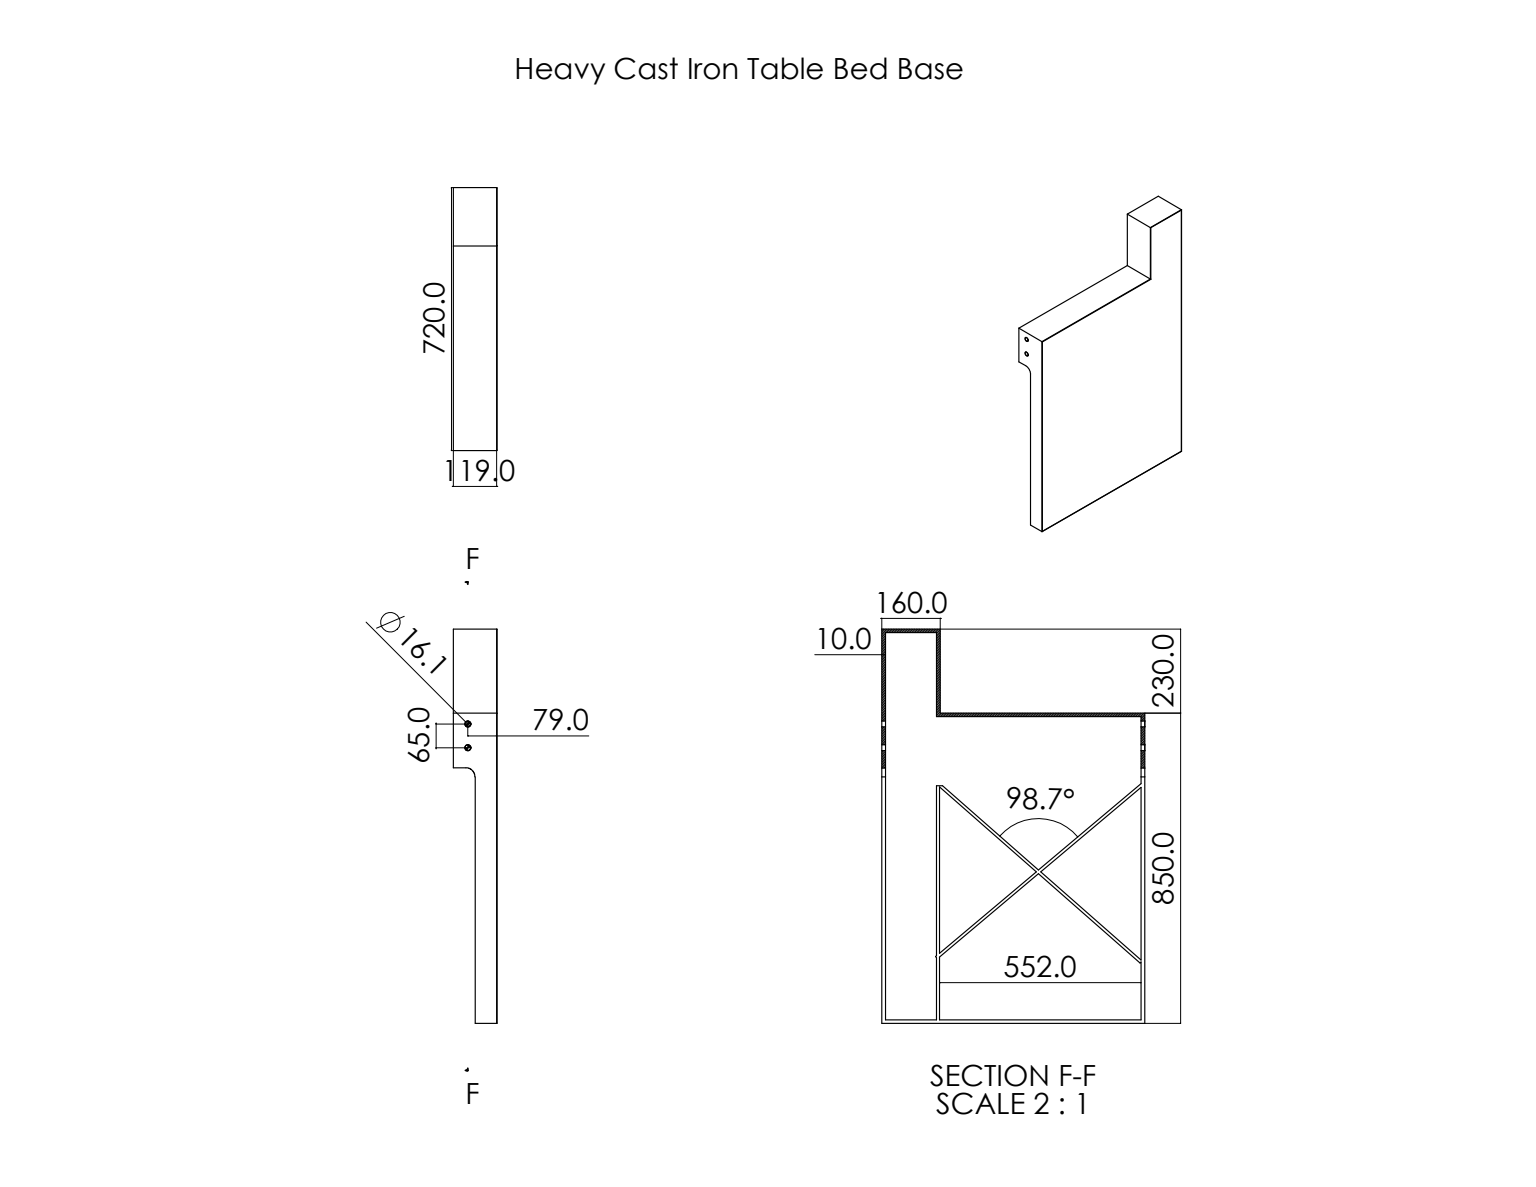
ISO-10303-21;
HEADER;
FILE_DESCRIPTION (('STEP AP214'),
    '1' );
FILE_NAME ('Heavy Cast Iron Table Bed Base.step',
    '2026-10-21T17:07:05',
    ( '' ),
    ( '' ),
    'SwSTEP 2.0',
    'SolidWorks 2025',
    '' );
FILE_SCHEMA (( 'AUTOMOTIVE_DESIGN' ));
ENDSEC;

DATA;
#65=ORIENTED_EDGE ( 'NONE', *, *, #36847, .T. ) ;
#80=ORIENTED_EDGE ( 'NONE', *, *, #38468, .F. ) ;
#82=DIRECTION ( 'NONE',  ( -0.000000000000000000, -1.000000000000000000, -0.000000000000000000 ) ) ;
#112=ORIENTED_EDGE ( 'NONE', *, *, #9772, .T. ) ;
#118=LINE ( 'NONE', #10283, #45262 ) ;
#145=CARTESIAN_POINT ( 'NONE',  ( 187.1337867209877857, 56.73212367640085318, 362.5753187112032379 ) ) ;
#155=DIRECTION ( 'NONE',  ( 0.000000000000000000, 0.000000000000000000, 1.000000000000000000 ) ) ;
#178=VECTOR ( 'NONE', #201, 1000.000000000000114 ) ;
#195=DIRECTION ( 'NONE',  ( 0.000000000000000000, -1.000000000000000000, 1.672022627447525240E-16 ) ) ;
#201=DIRECTION ( 'NONE',  ( -1.236450975029139710E-16, 0.7517448203044212462, 0.6594541114781782287 ) ) ;
#267=( BOUNDED_CURVE ( )  B_SPLINE_CURVE ( 3, ( #30983, #13892, #3032, #6720 ),
 .UNSPECIFIED., .F., .T. ) 
 B_SPLINE_CURVE_WITH_KNOTS ( ( 4, 4 ),
 ( 1.570796326794896558, 3.141592653589793116 ),
 .UNSPECIFIED. ) 
 CURVE ( )  GEOMETRIC_REPRESENTATION_ITEM ( )  RATIONAL_B_SPLINE_CURVE ( ( 1.000000000000000000, 0.8047378541243649375, 0.8047378541243649375, 1.000000000000000000 ) ) 
 REPRESENTATION_ITEM ( '' )  );
#273=CARTESIAN_POINT ( 'NONE',  ( 879.9999999999992042, 479.9999999999998863, -210.0000000000000000 ) ) ;
#291=AXIS2_PLACEMENT_3D ( 'NONE', #13040, #41443, #41905 ) ;
#352=EDGE_CURVE ( 'NONE', #861, #2741, #13234, .T. ) ;
#354=ORIENTED_EDGE ( 'NONE', *, *, #13193, .T. ) ;
#359=AXIS2_PLACEMENT_3D ( 'NONE', #31798, #9874, #27892 ) ;
#366=VECTOR ( 'NONE', #18473, 1000.000000000000000 ) ;
#377=DIRECTION ( 'NONE',  ( 0.000000000000000000, -0.6594541114781790059, 0.7517448203044204691 ) ) ;
#407=ORIENTED_EDGE ( 'NONE', *, *, #12306, .F. ) ;
#449=ADVANCED_FACE ( 'NONE', ( #27988 ), #38617, .F. ) ;
#535=EDGE_LOOP ( 'NONE', ( #2161, #41639, #39801, #23830 ) ) ;
#545=ORIENTED_EDGE ( 'NONE', *, *, #45289, .F. ) ;
#562=VECTOR ( 'NONE', #15359, 1000.000000000000000 ) ;
#623=DIRECTION ( 'NONE',  ( -0.000000000000000000, -0.000000000000000000, 1.000000000000000000 ) ) ;
#624=CARTESIAN_POINT ( 'NONE',  ( 999.9999999999992042, 239.9999999999998863, -209.9999999999999716 ) ) ;
#642=ORIENTED_EDGE ( 'NONE', *, *, #31723, .T. ) ;
#658=AXIS2_PLACEMENT_3D ( 'NONE', #4761, #18865, #32956 ) ;
#660=CARTESIAN_POINT ( 'NONE',  ( 989.9999999999992042, 62.79977829742938411, -207.3621835540872951 ) ) ;
#693=EDGE_CURVE ( 'NONE', #4054, #5516, #21293, .T. ) ;
#779=LINE ( 'NONE', #28956, #941 ) ;
#782=PLANE ( 'NONE',  #39472 ) ;
#802=CARTESIAN_POINT ( 'NONE',  ( 939.9999999999992042, 50.81038600091411439, -209.9999999999999716 ) ) ;
#826=DIRECTION ( 'NONE',  ( 1.000000000000000000, 0.000000000000000000, 0.000000000000000000 ) ) ;
#831=DIRECTION ( 'NONE',  ( 1.000000000000000000, -0.000000000000000000, 0.000000000000000000 ) ) ;
#849=EDGE_LOOP ( 'NONE', ( #8777, #12953, #44083, #25218 ) ) ;
#861=VERTEX_POINT ( 'NONE', #21514 ) ;
#884=( GEOMETRIC_REPRESENTATION_CONTEXT ( 3 ) GLOBAL_UNCERTAINTY_ASSIGNED_CONTEXT ( ( #29214 ) ) GLOBAL_UNIT_ASSIGNED_CONTEXT ( ( #30081, #19913, #9523 ) ) REPRESENTATION_CONTEXT ( 'NONE', 'WORKASPACE' ) );
#887=DIRECTION ( 'NONE',  ( 1.000000000000000000, -0.000000000000000000, -0.000000000000000000 ) ) ;
#920=EDGE_LOOP ( 'NONE', ( #2986, #31243, #45604, #112 ) ) ;
#937=CYLINDRICAL_SURFACE ( 'NONE', #26687, 1.000000000000000888 ) ;
#941=VECTOR ( 'NONE', #28498, 1000.000000000000000 ) ;
#960=EDGE_CURVE ( 'NONE', #27431, #8959, #32146, .T. ) ;
#966=VERTEX_POINT ( 'NONE', #41454 ) ;
#985=LINE ( 'NONE', #15090, #37294 ) ;
#1013=VECTOR ( 'NONE', #42593, 1000.000000000000000 ) ;
#1015=LINE ( 'NONE', #7286, #17369 ) ;
#1032=VERTEX_POINT ( 'NONE', #9806 ) ;
#1086=ORIENTED_EDGE ( 'NONE', *, *, #38685, .T. ) ;
#1104=DIRECTION ( 'NONE',  ( 0.000000000000000000, 0.7517448203044204691, 0.6594541114781790059 ) ) ;
#1115=AXIS2_PLACEMENT_3D ( 'NONE', #34295, #31290, #10275 ) ;
#1184=VECTOR ( 'NONE', #2168, 1000.000000000000000 ) ;
#1224=DIRECTION ( 'NONE',  ( -0.000000000000000000, -0.000000000000000000, -1.000000000000000000 ) ) ;
#1258=ADVANCED_FACE ( 'NONE', ( #30594 ), #30141, .T. ) ;
#1274=AXIS2_PLACEMENT_3D ( 'NONE', #17291, #20745, #24904 ) ;
#1308=CARTESIAN_POINT ( 'NONE',  ( 1820.038553321469863, -407.8586036264140375, -201.9999999999998863 ) ) ;
#1332=LINE ( 'NONE', #25597, #4420 ) ;
#1340=PLANE ( 'NONE',  #41833 ) ;
#1354=ORIENTED_EDGE ( 'NONE', *, *, #44887, .F. ) ;
#1358=LINE ( 'NONE', #15461, #15140 ) ;
#1397=CARTESIAN_POINT ( 'NONE',  ( 989.9999999999992042, 249.9999999999998863, 350.0000000000000000 ) ) ;
#1451=CARTESIAN_POINT ( 'NONE',  ( 914.9999999999992042, 99.99999999999984368, -350.0000000000000000 ) ) ;
#1463=FACE_OUTER_BOUND ( 'NONE', #20948, .T. ) ;
#1488=ORIENTED_EDGE ( 'NONE', *, *, #32844, .T. ) ;
#1513=DIRECTION ( 'NONE',  ( -1.058954862565134068E-16, 0.6438296778008191223, 0.7651688349527137056 ) ) ;
#1543=ADVANCED_FACE ( 'NONE', ( #10261 ), #24338, .F. ) ;
#1561=EDGE_CURVE ( 'NONE', #38354, #16465, #40038, .T. ) ;
#1599=EDGE_LOOP ( 'NONE', ( #39442, #9325, #33134, #32362 ) ) ;
#1601=DIRECTION ( 'NONE',  ( 0.000000000000000000, 0.7651688349527167032, -0.6438296778008156807 ) ) ;
#1678=CARTESIAN_POINT ( 'NONE',  ( 187.1337867209877857, -422.8782571739196783, -207.4246812887968190 ) ) ;
#1680=ORIENTED_EDGE ( 'NONE', *, *, #36506, .F. ) ;
#1729=( BOUNDED_CURVE ( )  B_SPLINE_CURVE ( 3, ( #32757, #8061, #36212, #40382 ),
 .UNSPECIFIED., .F., .T. ) 
 B_SPLINE_CURVE_WITH_KNOTS ( ( 4, 4 ),
 ( 4.712388980384689674, 6.283185307179586232 ),
 .UNSPECIFIED. ) 
 CURVE ( )  GEOMETRIC_REPRESENTATION_ITEM ( )  RATIONAL_B_SPLINE_CURVE ( ( 1.000000000000000000, 0.8047378541243649375, 0.8047378541243649375, 1.000000000000000000 ) ) 
 REPRESENTATION_ITEM ( '' )  );
#1751=AXIS2_PLACEMENT_3D ( 'NONE', #40538, #8887, #9347 ) ;
#1773=LINE ( 'NONE', #45441, #7634 ) ;
#1842=FACE_OUTER_BOUND ( 'NONE', #3408, .T. ) ;
#1846=EDGE_CURVE ( 'NONE', #22430, #39622, #19023, .T. ) ;
#1907=AXIS2_PLACEMENT_3D ( 'NONE', #37509, #40532, #8881 ) ;
#1920=DIRECTION ( 'NONE',  ( 1.000000000000000000, 0.000000000000000000, 0.000000000000000000 ) ) ;
#1935=DIRECTION ( 'NONE',  ( 0.000000000000000000, 0.000000000000000000, 1.000000000000000000 ) ) ;
#1941=ORIENTED_EDGE ( 'NONE', *, *, #25313, .F. ) ;
#1951=CARTESIAN_POINT ( 'NONE',  ( 999.9999999999992042, -600.0000000000001137, 359.0000000000000000 ) ) ;
#1973=CARTESIAN_POINT ( 'NONE',  ( 1820.038553321469863, -418.3138125091624602, -201.9999999999998863 ) ) ;
#1975=ORIENTED_EDGE ( 'NONE', *, *, #8593, .F. ) ;
#1989=ORIENTED_EDGE ( 'NONE', *, *, #19944, .T. ) ;
#2055=ORIENTED_EDGE ( 'NONE', *, *, #24398, .F. ) ;
#2059=FACE_BOUND ( 'NONE', #7636, .T. ) ;
#2079=EDGE_CURVE ( 'NONE', #40848, #12356, #33501, .T. ) ;
#2113=ORIENTED_EDGE ( 'NONE', *, *, #11760, .T. ) ;
#2156=ADVANCED_FACE ( 'NONE', ( #6514 ), #3046, .F. ) ;
#2157=ORIENTED_EDGE ( 'NONE', *, *, #14016, .F. ) ;
#2161=ORIENTED_EDGE ( 'NONE', *, *, #35912, .F. ) ;
#2168=DIRECTION ( 'NONE',  ( -0.000000000000000000, -0.000000000000000000, 1.000000000000000000 ) ) ;
#2197=LINE ( 'NONE', #41236, #38683 ) ;
#2201=CARTESIAN_POINT ( 'NONE',  ( 914.9999999999992042, 99.99999999999984368, 360.0000000000000000 ) ) ;
#2230=DIRECTION ( 'NONE',  ( 0.7071067811857625340, 0.000000000000000000, 0.7071067811873326114 ) ) ;
#2244=FACE_BOUND ( 'NONE', #18507, .T. ) ;
#2279=CARTESIAN_POINT ( 'NONE',  ( 989.9999999999992042, -590.0000000000001137, 360.0000000000000000 ) ) ;
#2345=DIRECTION ( 'NONE',  ( 1.000000000000000000, 0.000000000000000000, 0.000000000000000000 ) ) ;
#2365=ORIENTED_EDGE ( 'NONE', *, *, #4735, .T. ) ;
#2373=DIRECTION ( 'NONE',  ( 1.000000000000000000, 0.000000000000000000, -0.000000000000000000 ) ) ;
#2389=CARTESIAN_POINT ( 'NONE',  ( 939.9999999999993179, -590.0000000000001137, -209.9999999999999716 ) ) ;
#2407=VECTOR ( 'NONE', #30135, 1000.000000000000000 ) ;
#2444=ORIENTED_EDGE ( 'NONE', *, *, #21048, .F. ) ;
#2582=EDGE_CURVE ( 'NONE', #39622, #45702, #32793, .T. ) ;
#2584=LINE ( 'NONE', #16687, #20282 ) ;
#2611=CARTESIAN_POINT ( 'NONE',  ( 927.9999999999992042, 219.9999999999998863, -350.0000000000000000 ) ) ;
#2630=ADVANCED_FACE ( 'NONE', ( #36510 ), #4432, .T. ) ;
#2653=VECTOR ( 'NONE', #14168, 1000.000000000000000 ) ;
#2657=VECTOR ( 'NONE', #35418, 1000.000000000000000 ) ;
#2664=FACE_OUTER_BOUND ( 'NONE', #17522, .T. ) ;
#2693=CARTESIAN_POINT ( 'NONE',  ( 939.9999999999993179, -600.0000000000001137, -360.0000000000000000 ) ) ;
#2707=AXIS2_PLACEMENT_3D ( 'NONE', #35758, #1104, #14761 ) ;
#2741=VERTEX_POINT ( 'NONE', #23318 ) ;
#2742=ORIENTED_EDGE ( 'NONE', *, *, #25270, .T. ) ;
#2766=AXIS2_PLACEMENT_3D ( 'NONE', #23148, #37257, #2373 ) ;
#2826=LINE ( 'NONE', #36640, #40486 ) ;
#2830=DIRECTION ( 'NONE',  ( 0.000000000000000000, -1.000000000000000000, 0.000000000000000000 ) ) ;
#2888=DIRECTION ( 'NONE',  ( 0.000000000000000000, 0.000000000000000000, -1.000000000000000000 ) ) ;
#2960=ADVANCED_FACE ( 'NONE', ( #1842 ), #27635, .F. ) ;
#2986=ORIENTED_EDGE ( 'NONE', *, *, #41717, .T. ) ;
#2996=CARTESIAN_POINT ( 'NONE',  ( 914.9999999999992042, 74.99999999999984368, 350.0000000000000000 ) ) ;
#3032=CARTESIAN_POINT ( 'NONE',  ( 999.5857864376259840, 249.9999999999998863, -199.9999999999999432 ) ) ;
#3046=CYLINDRICAL_SURFACE ( 'NONE', #13598, 7.999999999999896083 ) ;
#3074=EDGE_LOOP ( 'NONE', ( #11565, #26546, #9323, #31356 ) ) ;
#3116=ORIENTED_EDGE ( 'NONE', *, *, #41125, .T. ) ;
#3147=DIRECTION ( 'NONE',  ( 0.000000000000000000, -1.000000000000000000, 0.000000000000000000 ) ) ;
#3183=ORIENTED_EDGE ( 'NONE', *, *, #16214, .F. ) ;
#3243=EDGE_LOOP ( 'NONE', ( #545, #41841, #11943 ) ) ;
#3252=ORIENTED_EDGE ( 'NONE', *, *, #8593, .T. ) ;
#3269=EDGE_CURVE ( 'NONE', #13352, #14381, #34673, .T. ) ;
#3311=AXIS2_PLACEMENT_3D ( 'NONE', #15950, #12699, #30032 ) ;
#3321=EDGE_LOOP ( 'NONE', ( #37502, #19598 ) ) ;
#3364=DIRECTION ( 'NONE',  ( 0.000000000000000000, 0.000000000000000000, 1.000000000000000000 ) ) ;
#3381=LINE ( 'NONE', #6608, #24751 ) ;
#3404=VECTOR ( 'NONE', #7997, 1000.000000000000000 ) ;
#3405=DIRECTION ( 'NONE',  ( -0.7071067811857625340, 8.659560562345319848E-17, 0.7071067811873326114 ) ) ;
#3408=EDGE_LOOP ( 'NONE', ( #13481, #19468, #22043, #26306 ) ) ;
#3413=FACE_OUTER_BOUND ( 'NONE', #849, .T. ) ;
#3424=CARTESIAN_POINT ( 'NONE',  ( 999.9999999999992042, -599.5857864376268935, -359.5857864376268935 ) ) ;
#3430=AXIS2_PLACEMENT_3D ( 'NONE', #8557, #4189, #19171 ) ;
#3548=ORIENTED_EDGE ( 'NONE', *, *, #352, .T. ) ;
#3573=EDGE_CURVE ( 'NONE', #13352, #40320, #25375, .T. ) ;
#3619=ORIENTED_EDGE ( 'NONE', *, *, #13436, .F. ) ;
#3663=PRODUCT_CONTEXT ( 'NONE', #30200, 'mechanical' ) ;
#3676=CARTESIAN_POINT ( 'NONE',  ( 939.9999999999992042, 62.85347435602262323, 357.4246812887967621 ) ) ;
#3723=DIRECTION ( 'NONE',  ( 1.000000000000000000, 0.000000000000000000, 0.000000000000000000 ) ) ;
#3779=CARTESIAN_POINT ( 'NONE',  ( 989.9999999999992042, 56.73212367640085318, 362.5753187112032379 ) ) ;
#3780=ORIENTED_EDGE ( 'NONE', *, *, #3573, .F. ) ;
#3791=FACE_BOUND ( 'NONE', #28122, .T. ) ;
#3846=CARTESIAN_POINT ( 'NONE',  ( 914.9999999999992042, 99.99999999999984368, -360.0000000000000000 ) ) ;
#3950=ADVANCED_FACE ( 'NONE', ( #22875 ), #36966, .T. ) ;
#3995=ORIENTED_EDGE ( 'NONE', *, *, #39851, .F. ) ;
#3999=CARTESIAN_POINT ( 'NONE',  ( 989.9999999999992042, 249.9999999999998863, 360.0000000000000000 ) ) ;
#4016=CARTESIAN_POINT ( 'NONE',  ( 914.9999999999992042, 74.99999999999984368, 360.0000000000000000 ) ) ;
#4029=AXIS2_PLACEMENT_3D ( 'NONE', #21182, #623, #4093 ) ;
#4038=CLOSED_SHELL ( 'NONE', ( #31058, #22434, #2960, #37465, #8867, #4331, #31468, #30827, #28338, #25562, #22339, #14811, #10351, #34267, #14270, #3950, #35401, #26673, #27265, #41594, #29738, #38511, #4476, #14559, #23886, #6850, #33445, #43897, #6939, #7678, #5215, #45345, #8096, #19314, #27472, #31110, #41238, #32888, #26409, #34218, #12002, #2156, #24657, #12343, #449, #30335, #30877, #12039, #2630, #42991, #19585, #31775, #1543, #29801, #26516, #34550, #24314, #17624, #43061, #1258 ) ) ;
#4054=VERTEX_POINT ( 'NONE', #7588 ) ;
#4066=AXIS2_PLACEMENT_3D ( 'NONE', #30420, #33670, #44059 ) ;
#4093=DIRECTION ( 'NONE',  ( 1.000000000000000000, 0.000000000000000000, 0.000000000000000000 ) ) ;
#4189=DIRECTION ( 'NONE',  ( -2.750100768424433062E-32, 1.672022627447525240E-16, 1.000000000000000000 ) ) ;
#4191=VECTOR ( 'NONE', #11167, 1000.000000000000114 ) ;
#4257=LINE ( 'NONE', #18348, #1013 ) ;
#4331=ADVANCED_FACE ( 'NONE', ( #8499 ), #20180, .F. ) ;
#4361=CARTESIAN_POINT ( 'NONE',  ( 989.9999999999992042, -590.0000000000001137, 360.0000000000000000 ) ) ;
#4364=FACE_OUTER_BOUND ( 'NONE', #3074, .T. ) ;
#4376=CARTESIAN_POINT ( 'NONE',  ( 879.9999999999990905, 479.9999999999998863, -360.0000000000000000 ) ) ;
#4399=VERTEX_POINT ( 'NONE', #16265 ) ;
#4407=ORIENTED_EDGE ( 'NONE', *, *, #14833, .F. ) ;
#4420=VECTOR ( 'NONE', #39707, 1000.000000000000000 ) ;
#4432=PLANE ( 'NONE',  #22454 ) ;
#4459=EDGE_LOOP ( 'NONE', ( #13895, #29449, #40745, #13582, #31975, #23501, #38647, #21754, #20248, #27040, #17573, #26011, #11888 ) ) ;
#4470=FACE_OUTER_BOUND ( 'NONE', #11164, .T. ) ;
#4476=ADVANCED_FACE ( 'NONE', ( #27345 ), #6329, .F. ) ;
#4494=PLANE ( 'NONE',  #23255 ) ;
#4623=CARTESIAN_POINT ( 'NONE',  ( 919.9999999999993179, 219.9999999999998863, 360.0000000000000000 ) ) ;
#4624=EDGE_CURVE ( 'NONE', #33095, #38247, #27804, .T. ) ;
#4646=CARTESIAN_POINT ( 'NONE',  ( 919.9999999999993179, 154.9999999999998863, 360.0000000000000000 ) ) ;
#4689=DIRECTION ( 'NONE',  ( 1.000000000000000000, 0.000000000000000000, -0.000000000000000000 ) ) ;
#4709=DIRECTION ( 'NONE',  ( -0.000000000000000000, -0.000000000000000000, 1.000000000000000000 ) ) ;
#4730=AXIS2_PLACEMENT_3D ( 'NONE', #23873, #5200, #37296 ) ;
#4735=EDGE_CURVE ( 'NONE', #23669, #34939, #13949, .T. ) ;
#4738=ORIENTED_EDGE ( 'NONE', *, *, #25587, .F. ) ;
#4740=DIRECTION ( 'NONE',  ( 0.000000000000000000, 0.000000000000000000, 1.000000000000000000 ) ) ;
#4761=CARTESIAN_POINT ( 'NONE',  ( 919.9999999999993179, 154.9999999999998863, -360.0000000000000000 ) ) ;
#4777=AXIS2_PLACEMENT_3D ( 'NONE', #19582, #20038, #34115 ) ;
#4785=VERTEX_POINT ( 'NONE', #32186 ) ;
#4874=DIRECTION ( 'NONE',  ( -0.000000000000000000, -0.000000000000000000, 1.000000000000000000 ) ) ;
#4887=EDGE_CURVE ( 'NONE', #966, #11789, #14409, .T. ) ;
#4932=AXIS2_PLACEMENT_3D ( 'NONE', #38324, #14069, #28141 ) ;
#4935=ORIENTED_EDGE ( 'NONE', *, *, #12607, .F. ) ;
#4952=ORIENTED_EDGE ( 'NONE', *, *, #25815, .F. ) ;
#4961=EDGE_LOOP ( 'NONE', ( #26851, #11042, #642, #17255 ) ) ;
#4995=EDGE_CURVE ( 'NONE', #16409, #17231, #985, .T. ) ;
#5034=CARTESIAN_POINT ( 'NONE',  ( 999.9999999999992042, -599.0000000000001137, 359.0000000000000000 ) ) ;
#5054=ORIENTED_EDGE ( 'NONE', *, *, #31723, .F. ) ;
#5077=ORIENTED_EDGE ( 'NONE', *, *, #5773, .F. ) ;
#5079=FACE_OUTER_BOUND ( 'NONE', #5281, .T. ) ;
#5085=EDGE_LOOP ( 'NONE', ( #40187, #7693 ) ) ;
#5147=CARTESIAN_POINT ( 'NONE',  ( -2.220446049250310809E-13, 479.9999999999994884, 0.000000000000000000 ) ) ;
#5176=EDGE_LOOP ( 'NONE', ( #31986, #24199, #30497 ) ) ;
#5200=DIRECTION ( 'NONE',  ( 0.000000000000000000, 0.000000000000000000, -1.000000000000000000 ) ) ;
#5201=DIRECTION ( 'NONE',  ( 1.000000000000000000, 0.000000000000000000, 0.000000000000000000 ) ) ;
#5215=ADVANCED_FACE ( 'NONE', ( #4470 ), #26380, .T. ) ;
#5237=CARTESIAN_POINT ( 'NONE',  ( 914.9999999999992042, 46.15097736693707020, 350.0000000000000000 ) ) ;
#5252=ORIENTED_EDGE ( 'NONE', *, *, #28896, .F. ) ;
#5281=EDGE_LOOP ( 'NONE', ( #26473, #28522, #9221, #12508 ) ) ;
#5401=PLANE ( 'NONE',  #1751 ) ;
#5406=CARTESIAN_POINT ( 'NONE',  ( 999.9999999999992042, 249.9999999999998863, -359.0000000000000000 ) ) ;
#5415=CARTESIAN_POINT ( 'NONE',  ( 919.9999999999993179, 219.9999999999998863, -360.0000000000000000 ) ) ;
#5443=EDGE_CURVE ( 'NONE', #24719, #9965, #23359, .T. ) ;
#5454=CYLINDRICAL_SURFACE ( 'NONE', #38766, 7.999999999999896083 ) ;
#5516=VERTEX_POINT ( 'NONE', #17773 ) ;
#5554=AXIS2_PLACEMENT_3D ( 'NONE', #25266, #25045, #28752 ) ;
#5560=VECTOR ( 'NONE', #5609, 1000.000000000000000 ) ;
#5609=DIRECTION ( 'NONE',  ( -1.000000000000000000, 0.000000000000000000, 0.000000000000000000 ) ) ;
#5639=CARTESIAN_POINT ( 'NONE',  ( 998.9999999999992042, 479.9999999999999432, -360.0000000000000000 ) ) ;
#5640=EDGE_LOOP ( 'NONE', ( #26576, #41313, #37034, #2113, #25208, #36979, #29286, #32303, #10113, #16109, #43701, #38019, #29087, #6247, #38707 ) ) ;
#5649=LINE ( 'NONE', #16275, #37778 ) ;
#5665=VECTOR ( 'NONE', #15441, 1000.000000000000000 ) ;
#5691=VERTEX_POINT ( 'NONE', #7601 ) ;
#5726=VECTOR ( 'NONE', #26797, 1000.000000000000000 ) ;
#5773=EDGE_CURVE ( 'NONE', #8959, #28228, #11068, .T. ) ;
#5805=ORIENTED_EDGE ( 'NONE', *, *, #19944, .F. ) ;
#5856=AXIS2_PLACEMENT_3D ( 'NONE', #23408, #8265, #11954 ) ;
#5857=ORIENTED_EDGE ( 'NONE', *, *, #6651, .T. ) ;
#5882=LINE ( 'NONE', #22959, #33402 ) ;
#5900=CARTESIAN_POINT ( 'NONE',  ( 989.9999999999992042, 469.9999999999999432, -350.0000000000000000 ) ) ;
#5939=PLANE ( 'NONE',  #43939 ) ;
#6072=ORIENTED_EDGE ( 'NONE', *, *, #4995, .T. ) ;
#6075=DIRECTION ( 'NONE',  ( 1.000000000000000000, 0.000000000000000000, 0.000000000000000000 ) ) ;
#6087=FACE_OUTER_BOUND ( 'NONE', #15314, .T. ) ;
#6121=PLANE ( 'NONE',  #1115 ) ;
#6128=CARTESIAN_POINT ( 'NONE',  ( 914.9999999999992042, 74.99999999999984368, -360.0000000000000000 ) ) ;
#6154=CARTESIAN_POINT ( 'NONE',  ( 879.9999999999990905, -414.5899773927342835, -210.0000000000000000 ) ) ;
#6160=ORIENTED_EDGE ( 'NONE', *, *, #25270, .F. ) ;
#6173=VECTOR ( 'NONE', #12244, 999.9999999999998863 ) ;
#6207=ORIENTED_EDGE ( 'NONE', *, *, #26420, .F. ) ;
#6221=CARTESIAN_POINT ( 'NONE',  ( 999.5857864376259840, 479.9999999999999432, -360.0000000000000000 ) ) ;
#6247=ORIENTED_EDGE ( 'NONE', *, *, #11400, .F. ) ;
#6255=VECTOR ( 'NONE', #44220, 1000.000000000000000 ) ;
#6272=AXIS2_PLACEMENT_3D ( 'NONE', #21978, #32598, #36284 ) ;
#6299=ORIENTED_EDGE ( 'NONE', *, *, #26147, .F. ) ;
#6306=DIRECTION ( 'NONE',  ( 0.000000000000000000, 0.000000000000000000, -1.000000000000000000 ) ) ;
#6307=VERTEX_POINT ( 'NONE', #31725 ) ;
#6329=PLANE ( 'NONE',  #35084 ) ;
#6361=AXIS2_PLACEMENT_3D ( 'NONE', #38757, #34597, #27897 ) ;
#6372=DIRECTION ( 'NONE',  ( 0.000000000000000000, -1.000000000000000000, 0.000000000000000000 ) ) ;
#6398=DIRECTION ( 'NONE',  ( -0.000000000000000000, -0.000000000000000000, 1.000000000000000000 ) ) ;
#6399=FACE_OUTER_BOUND ( 'NONE', #38480, .T. ) ;
#6404=CARTESIAN_POINT ( 'NONE',  ( 939.9999999999993179, -416.7569064942979935, -212.5753187112032947 ) ) ;
#6415=ORIENTED_EDGE ( 'NONE', *, *, #6651, .F. ) ;
#6453=DIRECTION ( 'NONE',  ( -0.000000000000000000, -0.000000000000000000, 1.000000000000000000 ) ) ;
#6487=CARTESIAN_POINT ( 'NONE',  ( 998.9999999999992042, 74.99999999999984368, -360.0000000000000000 ) ) ;
#6488=VERTEX_POINT ( 'NONE', #28037 ) ;
#6514=FACE_OUTER_BOUND ( 'NONE', #17073, .T. ) ;
#6542=ORIENTED_EDGE ( 'NONE', *, *, #40756, .F. ) ;
#6551=EDGE_CURVE ( 'NONE', #10806, #17231, #38671, .T. ) ;
#6608=CARTESIAN_POINT ( 'NONE',  ( 879.9999999999992042, 99.99999999999984368, -350.0000000000000000 ) ) ;
#6622=CARTESIAN_POINT ( 'NONE',  ( 989.9999999999992042, 62.79977829742938411, -207.3621835540872951 ) ) ;
#6651=EDGE_CURVE ( 'NONE', #40320, #16409, #18353, .T. ) ;
#6671=CARTESIAN_POINT ( 'NONE',  ( 928.0249999999991815, 154.9999999999998863, 360.0000000000000000 ) ) ;
#6720=CARTESIAN_POINT ( 'NONE',  ( 998.9999999999992042, 249.9999999999998863, -199.9999999999999716 ) ) ;
#6781=VECTOR ( 'NONE', #11345, 1000.000000000000114 ) ;
#6813=FACE_BOUND ( 'NONE', #43414, .T. ) ;
#6834=CIRCLE ( 'NONE', #35573, 7.999999999999896083 ) ;
#6837=CARTESIAN_POINT ( 'NONE',  ( 998.9999999999992042, 479.9999999999999432, -199.9999999999999716 ) ) ;
#6850=ADVANCED_FACE ( 'NONE', ( #25489, #3791, #22237 ), #782, .T. ) ;
#6892=DIRECTION ( 'NONE',  ( 0.000000000000000000, 0.000000000000000000, -1.000000000000000000 ) ) ;
#6905=EDGE_CURVE ( 'NONE', #23400, #8383, #28501, .T. ) ;
#6911=CARTESIAN_POINT ( 'NONE',  ( 998.9999999999992042, 479.9999999999999432, -360.0000000000000000 ) ) ;
#6921=EDGE_CURVE ( 'NONE', #11789, #11328, #40179, .T. ) ;
#6939=ADVANCED_FACE ( 'NONE', ( #30528 ), #36790, .T. ) ;
#7011=PLANE ( 'NONE',  #21086 ) ;
#7065=AXIS2_PLACEMENT_3D ( 'NONE', #32447, #39844, #32211 ) ;
#7074=CARTESIAN_POINT ( 'NONE',  ( 999.9999999999992042, 248.9999999999998863, 360.0000000000000000 ) ) ;
#7083=CIRCLE ( 'NONE', #1907, 24.99999999999991118 ) ;
#7085=CARTESIAN_POINT ( 'NONE',  ( 879.9999999999992042, 99.99999999999984368, 350.0000000000000000 ) ) ;
#7091=CIRCLE ( 'NONE', #12981, 7.999999999999896083 ) ;
#7112=ORIENTED_EDGE ( 'NONE', *, *, #39964, .F. ) ;
#7119=VECTOR ( 'NONE', #26208, 1000.000000000000114 ) ;
#7142=CARTESIAN_POINT ( 'NONE',  ( 939.9999999999994316, -428.4497686941065240, 352.6378164459125628 ) ) ;
#7185=EDGE_CURVE ( 'NONE', #25647, #34950, #26391, .T. ) ;
#7207=CARTESIAN_POINT ( 'NONE',  ( 939.9999999999992042, 56.73212367640090292, 362.5753187112032947 ) ) ;
#7268=CARTESIAN_POINT ( 'NONE',  ( 879.9999999999990905, 479.9999999999998863, -199.9999999999999716 ) ) ;
#7286=CARTESIAN_POINT ( 'NONE',  ( 187.1337867209877857, -179.7356316342496143, 69.11609595480014434 ) ) ;
#7322=CARTESIAN_POINT ( 'NONE',  ( 879.9999999999990905, 469.9999999999998863, -210.0000000000000000 ) ) ;
#7339=CARTESIAN_POINT ( 'NONE',  ( 911.9999999999993179, 154.9999999999998863, 360.0000000000000000 ) ) ;
#7343=DIRECTION ( 'NONE',  ( -0.000000000000000000, -0.000000000000000000, 1.000000000000000000 ) ) ;
#7459=ORIENTED_EDGE ( 'NONE', *, *, #16727, .F. ) ;
#7466=EDGE_LOOP ( 'NONE', ( #21881, #31490, #16621, #44658, #25867, #3116, #13071 ) ) ;
#7487=CARTESIAN_POINT ( 'NONE',  ( 914.9999999999990905, 469.9999999999999432, -350.0000000000000000 ) ) ;
#7556=DIRECTION ( 'NONE',  ( -1.084653538143406060E-16, 0.6594541114781790059, -0.7517448203044204691 ) ) ;
#7567=CARTESIAN_POINT ( 'NONE',  ( 998.9999999999992042, 249.9999999999998863, 360.0000000000000000 ) ) ;
#7588=CARTESIAN_POINT ( 'NONE',  ( 879.9999999999992042, 469.9999999999998863, -210.0000000000000000 ) ) ;
#7601=CARTESIAN_POINT ( 'NONE',  ( 914.9999999999992042, 99.99999999999984368, 360.0000000000000000 ) ) ;
#7620=ORIENTED_EDGE ( 'NONE', *, *, #8626, .T. ) ;
#7634=VECTOR ( 'NONE', #10539, 1000.000000000000000 ) ;
#7636=EDGE_LOOP ( 'NONE', ( #35810, #25110 ) ) ;
#7641=CARTESIAN_POINT ( 'NONE',  ( 879.9999999999990905, 479.9999999999998863, -360.0000000000000000 ) ) ;
#7658=EDGE_CURVE ( 'NONE', #9644, #41015, #2584, .T. ) ;
#7659=CARTESIAN_POINT ( 'NONE',  ( 914.9999999999992042, 74.99999999999984368, -350.0000000000000000 ) ) ;
#7667=CIRCLE ( 'NONE', #42340, 7.999999999999785061 ) ;
#7678=ADVANCED_FACE ( 'NONE', ( #15045 ), #14360, .T. ) ;
#7693=ORIENTED_EDGE ( 'NONE', *, *, #45012, .T. ) ;
#7723=VECTOR ( 'NONE', #25318, 1000.000000000000000 ) ;
#7733=ORIENTED_EDGE ( 'NONE', *, *, #21305, .F. ) ;
#7739=LINE ( 'NONE', #21586, #562 ) ;
#7766=CARTESIAN_POINT ( 'NONE',  ( 187.1337867209877857, 56.73212367640085318, 362.5753187112032379 ) ) ;
#7793=VECTOR ( 'NONE', #42146, 1000.000000000000000 ) ;
#7803=CARTESIAN_POINT ( 'NONE',  ( 989.9999999999992042, 56.60618624968560653, 350.0000000000000000 ) ) ;
#7829=EDGE_LOOP ( 'NONE', ( #19942, #40796, #21647, #32915, #37820, #44988, #44830 ) ) ;
#7851=VECTOR ( 'NONE', #32931, 1000.000000000000000 ) ;
#7873=ORIENTED_EDGE ( 'NONE', *, *, #4887, .F. ) ;
#7934=AXIS2_PLACEMENT_3D ( 'NONE', #14014, #30874, #34331 ) ;
#7957=DIRECTION ( 'NONE',  ( 1.000000000000000000, 0.000000000000000000, -0.000000000000000000 ) ) ;
#7992=EDGE_LOOP ( 'NONE', ( #3780, #19102, #5077, #31856, #16612, #5054, #3619 ) ) ;
#7997=DIRECTION ( 'NONE',  ( -1.337618101958019798E-16, 1.000000000000000000, -1.672022627447524747E-16 ) ) ;
#8033=CARTESIAN_POINT ( 'NONE',  ( 999.9999999999992042, 249.5857864376267798, 359.5857864376268935 ) ) ;
#8061=CARTESIAN_POINT ( 'NONE',  ( 999.9999999999992042, -599.5857864376268935, 359.5857864376268935 ) ) ;
#8096=ADVANCED_FACE ( 'NONE', ( #16395 ), #11810, .F. ) ;
#8129=DIRECTION ( 'NONE',  ( 0.000000000000000000, 0.7517448203044204691, 0.6594541114781790059 ) ) ;
#8132=FACE_OUTER_BOUND ( 'NONE', #13568, .T. ) ;
#8196=VERTEX_POINT ( 'NONE', #37872 ) ;
#8240=ORIENTED_EDGE ( 'NONE', *, *, #21048, .T. ) ;
#8265=DIRECTION ( 'NONE',  ( -1.000000000000000000, 0.000000000000000000, 0.000000000000000000 ) ) ;
#8269=PLANE ( 'NONE',  #2707 ) ;
#8292=LINE ( 'NONE', #18010, #15810 ) ;
#8301=EDGE_CURVE ( 'NONE', #4399, #40848, #44577, .T. ) ;
#8307=VERTEX_POINT ( 'NONE', #10154 ) ;
#8308=ORIENTED_EDGE ( 'NONE', *, *, #20723, .F. ) ;
#8323=EDGE_CURVE ( 'NONE', #12356, #8307, #16866, .T. ) ;
#8383=VERTEX_POINT ( 'NONE', #27024 ) ;
#8386=CARTESIAN_POINT ( 'NONE',  ( 989.9999999999992042, 50.81038600091411439, -193.6948738798775764 ) ) ;
#8408=LINE ( 'NONE', #40950, #10018 ) ;
#8416=DIRECTION ( 'NONE',  ( -0.000000000000000000, -0.000000000000000000, 1.000000000000000000 ) ) ;
#8499=FACE_OUTER_BOUND ( 'NONE', #23837, .T. ) ;
#8502=LINE ( 'NONE', #660, #14523 ) ;
#8505=DIRECTION ( 'NONE',  ( 0.000000000000000000, 0.000000000000000000, 1.000000000000000000 ) ) ;
#8557=CARTESIAN_POINT ( 'NONE',  ( 1820.038553321469863, 240.0000000000001990, -201.9999999999999716 ) ) ;
#8593=EDGE_CURVE ( 'NONE', #27904, #34950, #23464, .T. ) ;
#8617=VECTOR ( 'NONE', #42914, 1000.000000000000000 ) ;
#8624=PLANE ( 'NONE',  #26813 ) ;
#8626=EDGE_CURVE ( 'NONE', #28228, #42107, #22562, .T. ) ;
#8711=ORIENTED_EDGE ( 'NONE', *, *, #28285, .F. ) ;
#8777=ORIENTED_EDGE ( 'NONE', *, *, #33179, .F. ) ;
#8780=LINE ( 'NONE', #3779, #4191 ) ;
#8799=CARTESIAN_POINT ( 'NONE',  ( 999.9999999999992042, -599.0000000000001137, -359.0000000000000000 ) ) ;
#8835=VERTEX_POINT ( 'NONE', #44268 ) ;
#8858=CARTESIAN_POINT ( 'NONE',  ( 919.9999999999993179, 219.9999999999998863, -360.0000000000000000 ) ) ;
#8867=ADVANCED_FACE ( 'NONE', ( #22791 ), #5454, .F. ) ;
#8881=DIRECTION ( 'NONE',  ( 1.000000000000000000, 0.000000000000000000, 0.000000000000000000 ) ) ;
#8887=DIRECTION ( 'NONE',  ( 0.000000000000000000, 1.000000000000000000, -0.000000000000000000 ) ) ;
#8911=LINE ( 'NONE', #44242, #366 ) ;
#8942=DIRECTION ( 'NONE',  ( -1.000000000000000000, 0.000000000000000000, 0.000000000000000000 ) ) ;
#8959=VERTEX_POINT ( 'NONE', #2693 ) ;
#8964=CARTESIAN_POINT ( 'NONE',  ( 989.9999999999992042, -184.9457194955396631, 62.92409052808250891 ) ) ;
#8990=ORIENTED_EDGE ( 'NONE', *, *, #45289, .T. ) ;
#9066=CARTESIAN_POINT ( 'NONE',  ( 187.1337867209877857, -434.4637272565419153, 347.3621835540870961 ) ) ;
#9073=PRODUCT_DEFINITION_FORMATION_WITH_SPECIFIED_SOURCE ( 'ANY', '', #31792, .NOT_KNOWN. ) ;
#9074=LINE ( 'NONE', #26840, #5560 ) ;
#9085=ORIENTED_EDGE ( 'NONE', *, *, #30846, .F. ) ;
#9086=( NAMED_UNIT ( * ) SI_UNIT ( $, .STERADIAN. ) SOLID_ANGLE_UNIT ( ) );
#9128=CARTESIAN_POINT ( 'NONE',  ( 989.9999999999992042, -179.7356316342496712, 69.11609595480017276 ) ) ;
#9134=PLANE ( 'NONE',  #21787 ) ;
#9167=CARTESIAN_POINT ( 'NONE',  ( 939.9999999999993179, -422.8782571739196214, -207.4246812887968758 ) ) ;
#9170=CARTESIAN_POINT ( 'NONE',  ( 998.9999999999992042, -600.0000000000001137, 360.0000000000000000 ) ) ;
#9180=PLANE ( 'NONE',  #40076 ) ;
#9190=VECTOR ( 'NONE', #41087, 1000.000000000000000 ) ;
#9221=ORIENTED_EDGE ( 'NONE', *, *, #29530, .F. ) ;
#9244=VECTOR ( 'NONE', #30830, 1000.000000000000000 ) ;
#9293=VECTOR ( 'NONE', #30545, 1000.000000000000000 ) ;
#9323=ORIENTED_EDGE ( 'NONE', *, *, #9654, .T. ) ;
#9325=ORIENTED_EDGE ( 'NONE', *, *, #29475, .F. ) ;
#9338=PLANE ( 'NONE',  #5856 ) ;
#9347=DIRECTION ( 'NONE',  ( 0.000000000000000000, 0.000000000000000000, 1.000000000000000000 ) ) ;
#9356=VECTOR ( 'NONE', #8942, 1000.000000000000000 ) ;
#9417=DIRECTION ( 'NONE',  ( -1.000000000000000000, 2.412474565481389965E-32, -2.750100768424434704E-32 ) ) ;
#9444=( BOUNDED_CURVE ( )  B_SPLINE_CURVE ( 3, ( #6837, #27402, #27626, #45663 ),
 .UNSPECIFIED., .F., .T. ) 
 B_SPLINE_CURVE_WITH_KNOTS ( ( 4, 4 ),
 ( 0.000000000000000000, 1.570796326794896558 ),
 .UNSPECIFIED. ) 
 CURVE ( )  GEOMETRIC_REPRESENTATION_ITEM ( )  RATIONAL_B_SPLINE_CURVE ( ( 1.000000000000000000, 0.8047378541243649375, 0.8047378541243649375, 1.000000000000000000 ) ) 
 REPRESENTATION_ITEM ( '' )  );
#9506=ORIENTED_EDGE ( 'NONE', *, *, #10551, .F. ) ;
#9523=( NAMED_UNIT ( * ) SI_UNIT ( $, .STERADIAN. ) SOLID_ANGLE_UNIT ( ) );
#9595=CARTESIAN_POINT ( 'NONE',  ( 927.9999999999993179, 154.9999999999998863, 359.9749999999999659 ) ) ;
#9622=DIRECTION ( 'NONE',  ( -0.000000000000000000, -0.000000000000000000, 1.000000000000000000 ) ) ;
#9633=DIRECTION ( 'NONE',  ( 1.000000000000000000, 0.000000000000000000, 0.000000000000000000 ) ) ;
#9641=DIRECTION ( 'NONE',  ( 0.000000000000000000, -1.000000000000000000, 0.000000000000000000 ) ) ;
#9644=VERTEX_POINT ( 'NONE', #23407 ) ;
#9654=EDGE_CURVE ( 'NONE', #15578, #27431, #7083, .T. ) ;
#9659=EDGE_LOOP ( 'NONE', ( #4738, #36761, #26527, #41847 ) ) ;
#9732=CARTESIAN_POINT ( 'NONE',  ( 911.9999999999993179, 219.9999999999998863, 360.0000000000000000 ) ) ;
#9736=DIRECTION ( 'NONE',  ( 0.000000000000000000, 0.000000000000000000, 1.000000000000000000 ) ) ;
#9772=EDGE_CURVE ( 'NONE', #16409, #30556, #19267, .T. ) ;
#9786=CARTESIAN_POINT ( 'NONE',  ( 989.9999999999992042, 50.81038600091411439, -217.3872392842761769 ) ) ;
#9806=CARTESIAN_POINT ( 'NONE',  ( 939.9999999999993179, -600.0000000000001137, 360.0000000000000000 ) ) ;
#9829=ORIENTED_EDGE ( 'NONE', *, *, #28866, .F. ) ;
#9849=AXIS2_PLACEMENT_3D ( 'NONE', #20719, #7343, #21420 ) ;
#9850=DIRECTION ( 'NONE',  ( 1.000000000000000000, 0.000000000000000000, -0.000000000000000000 ) ) ;
#9860=LINE ( 'NONE', #31573, #14262 ) ;
#9864=DIRECTION ( 'NONE',  ( -0.000000000000000000, -0.000000000000000000, -1.000000000000000000 ) ) ;
#9874=DIRECTION ( 'NONE',  ( 4.625929269271485914E-16, -1.000000000000000000, 0.000000000000000000 ) ) ;
#9965=VERTEX_POINT ( 'NONE', #2389 ) ;
#10004=FACE_OUTER_BOUND ( 'NONE', #29565, .T. ) ;
#10018=VECTOR ( 'NONE', #26841, 1000.000000000000000 ) ;
#10026=CARTESIAN_POINT ( 'NONE',  ( 914.9999999999992042, 99.99999999999984368, 360.0000000000000000 ) ) ;
#10039=CARTESIAN_POINT ( 'NONE',  ( 998.9999999999992042, 479.9999999999998863, -199.9999999999999716 ) ) ;
#10057=LINE ( 'NONE', #24572, #32107 ) ;
#10060=ORIENTED_EDGE ( 'NONE', *, *, #11724, .F. ) ;
#10062=EDGE_CURVE ( 'NONE', #31920, #28192, #13945, .T. ) ;
#10089=DIRECTION ( 'NONE',  ( 1.000000000000000000, 0.000000000000000000, 0.000000000000000000 ) ) ;
#10113=ORIENTED_EDGE ( 'NONE', *, *, #960, .T. ) ;
#10154=CARTESIAN_POINT ( 'NONE',  ( 939.9999999999992042, 56.60618624968560653, 350.0000000000000000 ) ) ;
#10155=CARTESIAN_POINT ( 'NONE',  ( 999.9999999999992042, 479.5857864376268935, -359.5857864376268935 ) ) ;
#10188=DIRECTION ( 'NONE',  ( 1.337618101958019798E-16, -1.000000000000000000, 0.000000000000000000 ) ) ;
#10210=DIRECTION ( 'NONE',  ( 0.000000000000000000, -0.6438296778008192334, -0.7651688349527138167 ) ) ;
#10243=ORIENTED_EDGE ( 'NONE', *, *, #36032, .F. ) ;
#10246=LINE ( 'NONE', #20634, #15975 ) ;
#10250=CARTESIAN_POINT ( 'NONE',  ( 939.9999999999992042, 74.99999999999984368, -360.0000000000000000 ) ) ;
#10253=CARTESIAN_POINT ( 'NONE',  ( 939.9999999999992042, 47.45399382421949497, -201.9999999999999432 ) ) ;
#10261=FACE_OUTER_BOUND ( 'NONE', #19715, .T. ) ;
#10275=DIRECTION ( 'NONE',  ( -1.000000000000000000, 0.000000000000000000, -0.000000000000000000 ) ) ;
#10283=CARTESIAN_POINT ( 'NONE',  ( 989.9999999999992042, 249.9999999999998863, -209.9999999999999716 ) ) ;
#10310=LINE ( 'NONE', #7085, #34439 ) ;
#10323=CARTESIAN_POINT ( 'NONE',  ( 999.9999999999992042, 249.9999999999998863, -200.9999999999999432 ) ) ;
#10351=ADVANCED_FACE ( 'NONE', ( #25016 ), #7011, .T. ) ;
#10362=CARTESIAN_POINT ( 'NONE',  ( 999.9999999999992042, 248.9999999999998863, -200.9999999999999432 ) ) ;
#10379=DIRECTION ( 'NONE',  ( 0.000000000000000000, 0.000000000000000000, 1.000000000000000000 ) ) ;
#10390=EDGE_LOOP ( 'NONE', ( #40177, #25499, #16666, #24008, #19432, #34508 ) ) ;
#10411=LINE ( 'NONE', #20795, #16751 ) ;
#10468=CARTESIAN_POINT ( 'NONE',  ( 989.9999999999992042, 249.9999999999998863, 350.0000000000000000 ) ) ;
#10485=PLANE ( 'NONE',  #24624 ) ;
#10504=CARTESIAN_POINT ( 'NONE',  ( 939.9999999999993179, 62.79977829742944095, -207.3621835540873235 ) ) ;
#10539=DIRECTION ( 'NONE',  ( 1.644774851296528363E-16, -1.000000000000000000, 0.000000000000000000 ) ) ;
#10551=EDGE_CURVE ( 'NONE', #14381, #16198, #21100, .T. ) ;
#10559=LINE ( 'NONE', #44999, #26268 ) ;
#10689=ORIENTED_EDGE ( 'NONE', *, *, #12306, .T. ) ;
#10707=ORIENTED_EDGE ( 'NONE', *, *, #30371, .T. ) ;
#10711=CIRCLE ( 'NONE', #5554, 8.000000000000007105 ) ;
#10745=PLANE ( 'NONE',  #42291 ) ;
#10771=VECTOR ( 'NONE', #30569, 1000.000000000000000 ) ;
#10806=VERTEX_POINT ( 'NONE', #15991 ) ;
#10813=ORIENTED_EDGE ( 'NONE', *, *, #11170, .F. ) ;
#10848=VECTOR ( 'NONE', #34094, 1000.000000000000114 ) ;
#10938=ORIENTED_EDGE ( 'NONE', *, *, #27763, .F. ) ;
#10941=SHAPE_REPRESENTATION ( 'Heavy Cast Iron Table Bed Base', ( #26858 ), #39435 ) ;
#10960=DIRECTION ( 'NONE',  ( 0.000000000000000000, -1.000000000000000000, 1.672022627447524993E-16 ) ) ;
#11008=FACE_OUTER_BOUND ( 'NONE', #36046, .T. ) ;
#11041=EDGE_CURVE ( 'NONE', #42322, #23619, #16901, .T. ) ;
#11042=ORIENTED_EDGE ( 'NONE', *, *, #36032, .T. ) ;
#11060=CARTESIAN_POINT ( 'NONE',  ( 939.9999999999992042, -185.0721577059061929, 75.19946970736496894 ) ) ;
#11064=ORIENTED_EDGE ( 'NONE', *, *, #26420, .T. ) ;
#11068=LINE ( 'NONE', #25135, #13039 ) ;
#11104=CARTESIAN_POINT ( 'NONE',  ( 989.9999999999992042, -422.8782571739196783, -207.4246812887968190 ) ) ;
#11163=DIRECTION ( 'NONE',  ( -0.000000000000000000, -0.6438296778008192334, -0.7651688349527135946 ) ) ;
#11164=EDGE_LOOP ( 'NONE', ( #36484, #27374, #33300, #20784, #27661, #44663 ) ) ;
#11167=DIRECTION ( 'NONE',  ( -0.000000000000000000, -0.6438296778008192334, -0.7651688349527135946 ) ) ;
#11170=EDGE_CURVE ( 'NONE', #38205, #20464, #41385, .T. ) ;
#11244=CARTESIAN_POINT ( 'NONE',  ( 879.9999999999992042, 249.9999999999998295, 360.0000000000000000 ) ) ;
#11247=AXIS2_PLACEMENT_3D ( 'NONE', #15159, #32481, #35701 ) ;
#11259=EDGE_LOOP ( 'NONE', ( #10938, #17160, #3548, #39111 ) ) ;
#11280=LINE ( 'NONE', #32305, #5665 ) ;
#11317=DIRECTION ( 'NONE',  ( 0.000000000000000000, -1.000000000000000000, 0.000000000000000000 ) ) ;
#11328=VERTEX_POINT ( 'NONE', #14980 ) ;
#11345=DIRECTION ( 'NONE',  ( -1.058954862565134068E-16, 0.6438296778008191223, 0.7651688349527137056 ) ) ;
#11358=VECTOR ( 'NONE', #40549, 1000.000000000000114 ) ;
#11374=VECTOR ( 'NONE', #4689, 1000.000000000000000 ) ;
#11392=VERTEX_POINT ( 'NONE', #5034 ) ;
#11400=EDGE_CURVE ( 'NONE', #41469, #8307, #36213, .T. ) ;
#11418=FACE_OUTER_BOUND ( 'NONE', #535, .T. ) ;
#11419=DIRECTION ( 'NONE',  ( -1.000000000000000000, -4.625929269271485914E-16, 0.000000000000000000 ) ) ;
#11484=AXIS2_PLACEMENT_3D ( 'NONE', #45632, #38689, #31531 ) ;
#11486=LINE ( 'NONE', #7339, #37978 ) ;
#11501=ORIENTED_EDGE ( 'NONE', *, *, #7185, .F. ) ;
#11517=DIRECTION ( 'NONE',  ( 0.000000000000000000, -0.6594541114781790059, 0.7517448203044204691 ) ) ;
#11565=ORIENTED_EDGE ( 'NONE', *, *, #2582, .F. ) ;
#11571=CARTESIAN_POINT ( 'NONE',  ( 911.9749999999993406, 154.9999999999998863, 360.0000000000000000 ) ) ;
#11574=ORIENTED_EDGE ( 'NONE', *, *, #42141, .T. ) ;
#11584=CARTESIAN_POINT ( 'NONE',  ( 998.9999999999992042, 74.99999999999984368, 359.0000000000000000 ) ) ;
#11638=VECTOR ( 'NONE', #377, 1000.000000000000000 ) ;
#11675=VECTOR ( 'NONE', #20336, 1000.000000000000000 ) ;
#11683=EDGE_CURVE ( 'NONE', #24719, #16263, #35996, .T. ) ;
#11691=DIRECTION ( 'NONE',  ( -0.000000000000000000, -0.000000000000000000, 1.000000000000000000 ) ) ;
#11703=EDGE_CURVE ( 'NONE', #17901, #23619, #37805, .T. ) ;
#11708=LINE ( 'NONE', #624, #34579 ) ;
#11724=EDGE_CURVE ( 'NONE', #25647, #30052, #30186, .T. ) ;
#11750=CARTESIAN_POINT ( 'NONE',  ( 879.9999999999992042, 469.9999999999998863, 360.0000000000000000 ) ) ;
#11754=VERTEX_POINT ( 'NONE', #40595 ) ;
#11760=EDGE_CURVE ( 'NONE', #42322, #4785, #33420, .T. ) ;
#11789=VERTEX_POINT ( 'NONE', #43806 ) ;
#11795=DIRECTION ( 'NONE',  ( -0.000000000000000000, -0.000000000000000000, 1.000000000000000000 ) ) ;
#11810=PLANE ( 'NONE',  #17360 ) ;
#11856=CARTESIAN_POINT ( 'NONE',  ( 879.9999999999990905, 479.9999999999998863, -360.0000000000000000 ) ) ;
#11880=ORIENTED_EDGE ( 'NONE', *, *, #29475, .T. ) ;
#11888=ORIENTED_EDGE ( 'NONE', *, *, #4624, .T. ) ;
#11897=LINE ( 'NONE', #25071, #21851 ) ;
#11943=ORIENTED_EDGE ( 'NONE', *, *, #6905, .T. ) ;
#11954=DIRECTION ( 'NONE',  ( 0.000000000000000000, 0.000000000000000000, 1.000000000000000000 ) ) ;
#12002=ADVANCED_FACE ( 'NONE', ( #6399 ), #38723, .F. ) ;
#12005=EDGE_CURVE ( 'NONE', #41282, #4399, #10310, .T. ) ;
#12016=CARTESIAN_POINT ( 'NONE',  ( 914.9999999999992042, 99.99999999999984368, 350.0000000000000000 ) ) ;
#12039=ADVANCED_FACE ( 'NONE', ( #42180 ), #20482, .T. ) ;
#12117=ORIENTED_EDGE ( 'NONE', *, *, #27763, .T. ) ;
#12203=AXIS2_PLACEMENT_3D ( 'NONE', #22039, #35659, #17896 ) ;
#12229=AXIS2_PLACEMENT_3D ( 'NONE', #8858, #4709, #26177 ) ;
#12237=ORIENTED_EDGE ( 'NONE', *, *, #16989, .F. ) ;
#12244=DIRECTION ( 'NONE',  ( -0.7071067811857625340, 8.659560562345319848E-17, 0.7071067811873326114 ) ) ;
#12263=VECTOR ( 'NONE', #15245, 1000.000000000000000 ) ;
#12306=EDGE_CURVE ( 'NONE', #5691, #40848, #15155, .T. ) ;
#12322=EDGE_CURVE ( 'NONE', #30229, #41166, #21812, .T. ) ;
#12333=LINE ( 'NONE', #19704, #31411 ) ;
#12343=ADVANCED_FACE ( 'NONE', ( #11008 ), #18397, .T. ) ;
#12356=VERTEX_POINT ( 'NONE', #35468 ) ;
#12359=ORIENTED_EDGE ( 'NONE', *, *, #15433, .T. ) ;
#12386=CARTESIAN_POINT ( 'NONE',  ( 187.1337867209877857, 56.78581973499402835, -212.6378164459127049 ) ) ;
#12462=CARTESIAN_POINT ( 'NONE',  ( 989.9999999999992042, -590.0000000000001137, -209.9999999999999716 ) ) ;
#12508=ORIENTED_EDGE ( 'NONE', *, *, #31927, .F. ) ;
#12568=CARTESIAN_POINT ( 'NONE',  ( 999.9999999999992042, -600.0000000000001137, 360.0000000000000000 ) ) ;
#12607=EDGE_CURVE ( 'NONE', #42944, #10806, #11897, .T. ) ;
#12626=CARTESIAN_POINT ( 'NONE',  ( 919.9999999999993179, 154.9999999999998863, 360.0000000000000000 ) ) ;
#12699=DIRECTION ( 'NONE',  ( -0.000000000000000000, -0.000000000000000000, 1.000000000000000000 ) ) ;
#12717=CARTESIAN_POINT ( 'NONE',  ( 939.9999999999993179, 62.79977829742944095, -207.3621835540873235 ) ) ;
#12770=EDGE_LOOP ( 'NONE', ( #42336, #12117, #28889, #40301 ) ) ;
#12844=VERTEX_POINT ( 'NONE', #14470 ) ;
#12869=VECTOR ( 'NONE', #25020, 1000.000000000000000 ) ;
#12877=LINE ( 'NONE', #26962, #45140 ) ;
#12883=CIRCLE ( 'NONE', #4777, 7.999999999999896083 ) ;
#12901=LINE ( 'NONE', #26526, #43126 ) ;
#12906=EDGE_CURVE ( 'NONE', #11328, #24400, #36158, .T. ) ;
#12940=VECTOR ( 'NONE', #37098, 1000.000000000000000 ) ;
#12947=AXIS2_PLACEMENT_3D ( 'NONE', #7766, #32477, #21614 ) ;
#12953=ORIENTED_EDGE ( 'NONE', *, *, #12607, .T. ) ;
#12975=VECTOR ( 'NONE', #38906, 1000.000000000000000 ) ;
#12981=AXIS2_PLACEMENT_3D ( 'NONE', #36377, #4740, #18844 ) ;
#13007=LINE ( 'NONE', #34009, #35834 ) ;
#13024=ORIENTED_EDGE ( 'NONE', *, *, #28401, .T. ) ;
#13039=VECTOR ( 'NONE', #887, 1000.000000000000000 ) ;
#13040=CARTESIAN_POINT ( 'NONE',  ( 879.9999999999990905, 479.9999999999998863, -210.0000000000000000 ) ) ;
#13055=FACE_OUTER_BOUND ( 'NONE', #39289, .T. ) ;
#13071=ORIENTED_EDGE ( 'NONE', *, *, #40816, .T. ) ;
#13086=EDGE_CURVE ( 'NONE', #37952, #41015, #7091, .T. ) ;
#13108=CARTESIAN_POINT ( 'NONE',  ( 919.9999999999993179, 219.9999999999998863, -350.0000000000000000 ) ) ;
#13193=EDGE_CURVE ( 'NONE', #17901, #29615, #40983, .T. ) ;
#13207=ORIENTED_EDGE ( 'NONE', *, *, #19682, .F. ) ;
#13234=LINE ( 'NONE', #9066, #34288 ) ;
#13249=CARTESIAN_POINT ( 'NONE',  ( 998.9999999999992042, 248.9999999999998863, 360.0000000000000000 ) ) ;
#13294=PLANE ( 'NONE',  #12203 ) ;
#13352=VERTEX_POINT ( 'NONE', #5639 ) ;
#13380=DIRECTION ( 'NONE',  ( -0.000000000000000000, -0.000000000000000000, -1.000000000000000000 ) ) ;
#13425=VECTOR ( 'NONE', #3405, 999.9999999999998863 ) ;
#13436=EDGE_CURVE ( 'NONE', #40320, #25938, #20855, .T. ) ;
#13481=ORIENTED_EDGE ( 'NONE', *, *, #6921, .F. ) ;
#13483=ORIENTED_EDGE ( 'NONE', *, *, #15671, .F. ) ;
#13493=ORIENTED_EDGE ( 'NONE', *, *, #32811, .T. ) ;
#13551=EDGE_CURVE ( 'NONE', #28289, #4399, #10246, .T. ) ;
#13554=DIRECTION ( 'NONE',  ( 0.000000000000000000, -0.6438296778008192334, -0.7651688349527138167 ) ) ;
#13568=EDGE_LOOP ( 'NONE', ( #29071, #26926, #30510, #6299 ) ) ;
#13569=AXIS2_PLACEMENT_3D ( 'NONE', #24558, #38674, #18574 ) ;
#13582=ORIENTED_EDGE ( 'NONE', *, *, #31883, .F. ) ;
#13598=AXIS2_PLACEMENT_3D ( 'NONE', #41399, #42298, #17367 ) ;
#13643=DIRECTION ( 'NONE',  ( -0.000000000000000000, -0.000000000000000000, 1.000000000000000000 ) ) ;
#13695=VERTEX_POINT ( 'NONE', #45603 ) ;
#13707=ORIENTED_EDGE ( 'NONE', *, *, #8301, .T. ) ;
#13719=CIRCLE ( 'NONE', #12229, 7.999999999999785061 ) ;
#13783=CARTESIAN_POINT ( 'NONE',  ( 989.9999999999992042, 47.45399382421947365, -201.9999999999999432 ) ) ;
#13814=PLANE ( 'NONE',  #15104 ) ;
#13851=AXIS2_PLACEMENT_3D ( 'NONE', #43906, #44134, #26359 ) ;
#13892=CARTESIAN_POINT ( 'NONE',  ( 999.9999999999992042, 249.5857864376267798, -200.4142135623730496 ) ) ;
#13895=ORIENTED_EDGE ( 'NONE', *, *, #25313, .T. ) ;
#13945=LINE ( 'NONE', #9786, #10771 ) ;
#13949=LINE ( 'NONE', #24789, #12975 ) ;
#14014=CARTESIAN_POINT ( 'NONE',  ( 998.9999999999992042, 249.9999999999998863, -200.9999999999999432 ) ) ;
#14016=EDGE_CURVE ( 'NONE', #33479, #38417, #8780, .T. ) ;
#14020=CARTESIAN_POINT ( 'NONE',  ( 989.9999999999992042, -185.0721577059061929, 75.19946970736501157 ) ) ;
#14052=VERTEX_POINT ( 'NONE', #32424 ) ;
#14069=DIRECTION ( 'NONE',  ( -0.000000000000000000, -0.000000000000000000, -1.000000000000000000 ) ) ;
#14159=EDGE_LOOP ( 'NONE', ( #23110, #31541, #26844, #24065 ) ) ;
#14168=DIRECTION ( 'NONE',  ( -0.000000000000000000, -0.000000000000000000, 1.000000000000000000 ) ) ;
#14171=EDGE_LOOP ( 'NONE', ( #42328, #23959, #32172, #29110 ) ) ;
#14175=VERTEX_POINT ( 'NONE', #30455 ) ;
#14227=EDGE_CURVE ( 'NONE', #37975, #44323, #41328, .T. ) ;
#14262=VECTOR ( 'NONE', #28313, 1000.000000000000227 ) ;
#14270=ADVANCED_FACE ( 'NONE', ( #33710, #2059, #16152 ), #40866, .F. ) ;
#14289=CARTESIAN_POINT ( 'NONE',  ( 879.9999999999990905, -419.8175818341089780, -210.0000000000000000 ) ) ;
#14290=DIRECTION ( 'NONE',  ( -0.000000000000000000, -0.000000000000000000, 1.000000000000000000 ) ) ;
#14360=PLANE ( 'NONE',  #6272 ) ;
#14381=VERTEX_POINT ( 'NONE', #34837 ) ;
#14409=LINE ( 'NONE', #34726, #12869 ) ;
#14447=CARTESIAN_POINT ( 'NONE',  ( 911.9999999999992042, 154.9999999999998863, 359.9749999999999659 ) ) ;
#14449=VERTEX_POINT ( 'NONE', #11060 ) ;
#14470=CARTESIAN_POINT ( 'NONE',  ( 989.9999999999992042, 240.0000000000000568, -210.0000000000000000 ) ) ;
#14482=VECTOR ( 'NONE', #32473, 999.9999999999998863 ) ;
#14486=LINE ( 'NONE', #28566, #18745 ) ;
#14523=VECTOR ( 'NONE', #11517, 1000.000000000000000 ) ;
#14559=ADVANCED_FACE ( 'NONE', ( #17539 ), #24216, .F. ) ;
#14632=CARTESIAN_POINT ( 'NONE',  ( 939.9999999999993179, -590.0000000000001137, -201.9999999999998579 ) ) ;
#14633=ORIENTED_EDGE ( 'NONE', *, *, #32926, .T. ) ;
#14649=EDGE_LOOP ( 'NONE', ( #32184, #23487, #38137, #21874, #43689, #32856, #21893 ) ) ;
#14655=CIRCLE ( 'NONE', #45607, 8.024999999999948841 ) ;
#14675=CARTESIAN_POINT ( 'NONE',  ( 919.9999999999993179, 219.9999999999998863, 360.0000000000000000 ) ) ;
#14746=ORIENTED_EDGE ( 'NONE', *, *, #7185, .T. ) ;
#14761=DIRECTION ( 'NONE',  ( 0.000000000000000000, -0.6594541114781790059, 0.7517448203044204691 ) ) ;
#14790=ORIENTED_EDGE ( 'NONE', *, *, #39431, .F. ) ;
#14811=ADVANCED_FACE ( 'NONE', ( #18671 ), #1340, .T. ) ;
#14833=EDGE_CURVE ( 'NONE', #19176, #4054, #43382, .T. ) ;
#14869=CARTESIAN_POINT ( 'NONE',  ( 999.9999999999992042, 478.9999999999999432, -199.9999999999999716 ) ) ;
#14925=PLANE ( 'NONE',  #34448 ) ;
#14980=CARTESIAN_POINT ( 'NONE',  ( 927.9999999999993179, 219.9999999999998863, 359.9749999999999659 ) ) ;
#15008=ORIENTED_EDGE ( 'NONE', *, *, #26387, .F. ) ;
#15045=FACE_OUTER_BOUND ( 'NONE', #17514, .T. ) ;
#15090=CARTESIAN_POINT ( 'NONE',  ( 879.9999999999990905, 479.9999999999998863, -199.9999999999999716 ) ) ;
#15097=DIRECTION ( 'NONE',  ( -1.000000000000000000, -4.625929269271485914E-16, 0.000000000000000000 ) ) ;
#15104=AXIS2_PLACEMENT_3D ( 'NONE', #38508, #44994, #38294 ) ;
#15131=VECTOR ( 'NONE', #27702, 1000.000000000000000 ) ;
#15140=VECTOR ( 'NONE', #29539, 1000.000000000000000 ) ;
#15155=LINE ( 'NONE', #21395, #26230 ) ;
#15159=CARTESIAN_POINT ( 'NONE',  ( 919.9999999999993179, 154.9999999999998863, 359.9749999999999659 ) ) ;
#15160=FACE_OUTER_BOUND ( 'NONE', #11259, .T. ) ;
#15226=ORIENTED_EDGE ( 'NONE', *, *, #41564, .T. ) ;
#15245=DIRECTION ( 'NONE',  ( -0.000000000000000000, -0.000000000000000000, 1.000000000000000000 ) ) ;
#15269=DIRECTION ( 'NONE',  ( 1.000000000000000000, 0.000000000000000000, 0.000000000000000000 ) ) ;
#15272=EDGE_LOOP ( 'NONE', ( #34038, #7620, #45226, #44553 ) ) ;
#15310=ORIENTED_EDGE ( 'NONE', *, *, #28382, .T. ) ;
#15314=EDGE_LOOP ( 'NONE', ( #11064, #9506, #28707, #7733 ) ) ;
#15350=CARTESIAN_POINT ( 'NONE',  ( 879.9999999999990905, 479.9999999999998863, -210.0000000000000000 ) ) ;
#15359=DIRECTION ( 'NONE',  ( 0.000000000000000000, -1.000000000000000000, 0.000000000000000000 ) ) ;
#15433=EDGE_CURVE ( 'NONE', #15624, #25647, #34788, .T. ) ;
#15441=DIRECTION ( 'NONE',  ( 1.337618101958019798E-16, -1.000000000000000000, 0.000000000000000000 ) ) ;
#15461=CARTESIAN_POINT ( 'NONE',  ( 998.9999999999992042, 249.9999999999998863, 360.0000000000000000 ) ) ;
#15501=LINE ( 'NONE', #1397, #18570 ) ;
#15569=FACE_OUTER_BOUND ( 'NONE', #26989, .T. ) ;
#15573=ORIENTED_EDGE ( 'NONE', *, *, #5443, .F. ) ;
#15578=VERTEX_POINT ( 'NONE', #3846 ) ;
#15624=VERTEX_POINT ( 'NONE', #14020 ) ;
#15647=DIRECTION ( 'NONE',  ( -1.000000000000000000, 0.000000000000000000, 0.000000000000000000 ) ) ;
#15654=EDGE_CURVE ( 'NONE', #4054, #25632, #20485, .T. ) ;
#15671=EDGE_CURVE ( 'NONE', #34011, #31920, #18852, .T. ) ;
#15685=ORIENTED_EDGE ( 'NONE', *, *, #45012, .F. ) ;
#15782=DIRECTION ( 'NONE',  ( 0.000000000000000000, -0.6438296778008156807, -0.7651688349527167032 ) ) ;
#15810=VECTOR ( 'NONE', #22144, 1000.000000000000000 ) ;
#15850=CIRCLE ( 'NONE', #39489, 7.999999999999896083 ) ;
#15895=CARTESIAN_POINT ( 'NONE',  ( 1820.038553321469863, -589.9999999999998863, -201.9999999999998579 ) ) ;
#15902=VERTEX_POINT ( 'NONE', #43539 ) ;
#15946=EDGE_CURVE ( 'NONE', #34100, #20728, #18601, .T. ) ;
#15950=CARTESIAN_POINT ( 'NONE',  ( 919.9999999999993179, 219.9999999999998863, 360.0000000000000000 ) ) ;
#15969=FACE_OUTER_BOUND ( 'NONE', #22160, .T. ) ;
#15975=VECTOR ( 'NONE', #31264, 1000.000000000000000 ) ;
#15991=CARTESIAN_POINT ( 'NONE',  ( 998.9999999999992042, 249.9999999999998863, -199.9999999999999716 ) ) ;
#16004=CARTESIAN_POINT ( 'NONE',  ( 914.9999999999992042, 74.99999999999984368, 350.0000000000000000 ) ) ;
#16017=DIRECTION ( 'NONE',  ( 1.000000000000000000, -0.000000000000000000, -0.000000000000000000 ) ) ;
#16052=DIRECTION ( 'NONE',  ( 1.000000000000000000, 0.000000000000000000, 0.000000000000000000 ) ) ;
#16109=ORIENTED_EDGE ( 'NONE', *, *, #29187, .F. ) ;
#16152=FACE_OUTER_BOUND ( 'NONE', #14649, .T. ) ;
#16194=EDGE_CURVE ( 'NONE', #11328, #11789, #36291, .T. ) ;
#16198=VERTEX_POINT ( 'NONE', #27134 ) ;
#16211=EDGE_CURVE ( 'NONE', #38247, #41282, #5649, .T. ) ;
#16214=EDGE_CURVE ( 'NONE', #37728, #14381, #37522, .T. ) ;
#16263=VERTEX_POINT ( 'NONE', #30584 ) ;
#16265=CARTESIAN_POINT ( 'NONE',  ( 879.9999999999992042, 99.99999999999984368, 350.0000000000000000 ) ) ;
#16275=CARTESIAN_POINT ( 'NONE',  ( 999.9999999999992042, 239.9999999999998863, 350.0000000000000000 ) ) ;
#16370=VECTOR ( 'NONE', #23181, 1000.000000000000000 ) ;
#16395=FACE_OUTER_BOUND ( 'NONE', #18483, .T. ) ;
#16409=VERTEX_POINT ( 'NONE', #7268 ) ;
#16445=DIRECTION ( 'NONE',  ( 0.000000000000000000, 1.000000000000000000, -0.000000000000000000 ) ) ;
#16462=CARTESIAN_POINT ( 'NONE',  ( 989.9999999999992042, 249.9999999999998863, -350.0000000000000000 ) ) ;
#16465=VERTEX_POINT ( 'NONE', #10253 ) ;
#16477=( LENGTH_UNIT ( ) NAMED_UNIT ( * ) SI_UNIT ( .MILLI., .METRE. ) );
#16482=ORIENTED_EDGE ( 'NONE', *, *, #13551, .T. ) ;
#16530=ORIENTED_EDGE ( 'NONE', *, *, #21305, .T. ) ;
#16553=DIRECTION ( 'NONE',  ( 0.000000000000000000, -1.000000000000000000, 0.000000000000000000 ) ) ;
#16576=DIRECTION ( 'NONE',  ( -1.000000000000000000, 0.000000000000000000, -0.000000000000000000 ) ) ;
#16602=CARTESIAN_POINT ( 'NONE',  ( 999.5857864376259840, -600.0000000000001137, -360.0000000000000000 ) ) ;
#16612=ORIENTED_EDGE ( 'NONE', *, *, #9654, .F. ) ;
#16621=ORIENTED_EDGE ( 'NONE', *, *, #33179, .T. ) ;
#16666=ORIENTED_EDGE ( 'NONE', *, *, #16214, .T. ) ;
#16687=CARTESIAN_POINT ( 'NONE',  ( 927.9999999999992042, 154.9999999999998863, 360.0000000000000000 ) ) ;
#16727=EDGE_CURVE ( 'NONE', #6488, #12356, #41447, .T. ) ;
#16748=CARTESIAN_POINT ( 'NONE',  ( 939.9999999999993179, -600.0000000000001137, -360.0000000000000000 ) ) ;
#16751=VECTOR ( 'NONE', #10188, 1000.000000000000000 ) ;
#16866=LINE ( 'NONE', #34157, #15131 ) ;
#16901=LINE ( 'NONE', #3676, #21882 ) ;
#16939=CYLINDRICAL_SURFACE ( 'NONE', #25619, 1.000000000000000888 ) ;
#16989=EDGE_CURVE ( 'NONE', #28289, #5691, #779, .T. ) ;
#17019=DIRECTION ( 'NONE',  ( 1.000000000000000000, 4.625929269271485914E-16, 0.000000000000000000 ) ) ;
#17027=EDGE_CURVE ( 'NONE', #30441, #19176, #39137, .T. ) ;
#17030=CARTESIAN_POINT ( 'NONE',  ( 879.9999999999992042, 99.99999999999984368, 360.0000000000000000 ) ) ;
#17045=ORIENTED_EDGE ( 'NONE', *, *, #23279, .F. ) ;
#17067=CARTESIAN_POINT ( 'NONE',  ( 989.9999999999992042, 239.9999999999998863, 360.0000000000000000 ) ) ;
#17073=EDGE_LOOP ( 'NONE', ( #10813, #31702, #33636, #11574 ) ) ;
#17160=ORIENTED_EDGE ( 'NONE', *, *, #41564, .F. ) ;
#17180=FACE_OUTER_BOUND ( 'NONE', #29062, .T. ) ;
#17219=MANIFOLD_SOLID_BREP ( 'Fillet2', #4038 ) ;
#17223=CIRCLE ( 'NONE', #21646, 24.99999999999991118 ) ;
#17231=VERTEX_POINT ( 'NONE', #26157 ) ;
#17255=ORIENTED_EDGE ( 'NONE', *, *, #21883, .F. ) ;
#17260=LINE ( 'NONE', #27652, #26166 ) ;
#17291=CARTESIAN_POINT ( 'NONE',  ( 914.9999999999992042, 74.99999999999984368, 350.0000000000000000 ) ) ;
#17292=CARTESIAN_POINT ( 'NONE',  ( 927.9999999999992042, 154.9999999999998863, -350.0000000000000000 ) ) ;
#17322=VECTOR ( 'NONE', #25928, 1000.000000000000000 ) ;
#17360=AXIS2_PLACEMENT_3D ( 'NONE', #2996, #20310, #31164 ) ;
#17367=DIRECTION ( 'NONE',  ( 1.000000000000000000, 0.000000000000000000, 0.000000000000000000 ) ) ;
#17369=VECTOR ( 'NONE', #43287, 1000.000000000000000 ) ;
#17376=VECTOR ( 'NONE', #42145, 1000.000000000000000 ) ;
#17397=VERTEX_POINT ( 'NONE', #42071 ) ;
#17443=CARTESIAN_POINT ( 'NONE',  ( 919.9999999999993179, 154.9999999999998863, 350.0000000000000000 ) ) ;
#17511=FACE_OUTER_BOUND ( 'NONE', #1599, .T. ) ;
#17514=EDGE_LOOP ( 'NONE', ( #39749, #1941, #45221, #43559 ) ) ;
#17522=EDGE_LOOP ( 'NONE', ( #12359, #14746, #42525 ) ) ;
#17539=FACE_OUTER_BOUND ( 'NONE', #20045, .T. ) ;
#17557=CARTESIAN_POINT ( 'NONE',  ( 989.9999999999992042, -418.3138125091626307, -201.9999999999998010 ) ) ;
#17573=ORIENTED_EDGE ( 'NONE', *, *, #25815, .T. ) ;
#17591=CARTESIAN_POINT ( 'NONE',  ( 989.9999999999992042, 469.9999999999999432, 360.0000000000000000 ) ) ;
#17624=ADVANCED_FACE ( 'NONE', ( #17821 ), #937, .T. ) ;
#17642=EDGE_CURVE ( 'NONE', #14449, #27904, #25185, .T. ) ;
#17643=VECTOR ( 'NONE', #25433, 1000.000000000000114 ) ;
#17653=CARTESIAN_POINT ( 'NONE',  ( 879.9999999999992042, 99.99999999999984368, -360.0000000000000000 ) ) ;
#17740=LINE ( 'NONE', #20509, #40303 ) ;
#17773=CARTESIAN_POINT ( 'NONE',  ( 879.9999999999992042, 239.9999999999998295, -210.0000000000000000 ) ) ;
#17791=ORIENTED_EDGE ( 'NONE', *, *, #28721, .F. ) ;
#17821=FACE_OUTER_BOUND ( 'NONE', #26584, .T. ) ;
#17866=EDGE_CURVE ( 'NONE', #37975, #8835, #15501, .T. ) ;
#17871=ORIENTED_EDGE ( 'NONE', *, *, #11703, .F. ) ;
#17896=DIRECTION ( 'NONE',  ( 0.000000000000000000, 0.000000000000000000, 1.000000000000000000 ) ) ;
#17901=VERTEX_POINT ( 'NONE', #22398 ) ;
#17973=SHAPE_DEFINITION_REPRESENTATION ( #44674, #10941 ) ;
#18010=CARTESIAN_POINT ( 'NONE',  ( 939.9999999999993179, -600.0000000000001137, 360.0000000000000000 ) ) ;
#18058=AXIS2_PLACEMENT_3D ( 'NONE', #5147, #40275, #26160 ) ;
#18111=DIRECTION ( 'NONE',  ( 1.000000000000000000, 0.000000000000000000, -0.000000000000000000 ) ) ;
#18126=DIRECTION ( 'NONE',  ( 1.000000000000000000, 0.000000000000000000, 0.000000000000000000 ) ) ;
#18133=CARTESIAN_POINT ( 'NONE',  ( 879.9999999999992042, 99.99999999999984368, -350.0000000000000000 ) ) ;
#18153=APPLICATION_CONTEXT ( 'automotive_design' ) ;
#18184=CIRCLE ( 'NONE', #6361, 7.999999999999896083 ) ;
#18335=ORIENTED_EDGE ( 'NONE', *, *, #15654, .T. ) ;
#18340=LINE ( 'NONE', #25235, #40368 ) ;
#18347=VECTOR ( 'NONE', #9864, 1000.000000000000000 ) ;
#18348=CARTESIAN_POINT ( 'NONE',  ( 999.9999999999992042, -600.0000000000001137, 360.0000000000000000 ) ) ;
#18353=LINE ( 'NONE', #11856, #17322 ) ;
#18381=ORIENTED_EDGE ( 'NONE', *, *, #36740, .F. ) ;
#18397=PLANE ( 'NONE',  #12947 ) ;
#18466=DIRECTION ( 'NONE',  ( -1.000000000000000000, -4.625929269271485914E-16, -0.000000000000000000 ) ) ;
#18473=DIRECTION ( 'NONE',  ( -0.000000000000000000, -0.000000000000000000, -1.000000000000000000 ) ) ;
#18483=EDGE_LOOP ( 'NONE', ( #11501, #24542, #43974, #3252 ) ) ;
#18489=LINE ( 'NONE', #39748, #39450 ) ;
#18490=ORIENTED_EDGE ( 'NONE', *, *, #31734, .F. ) ;
#18507=EDGE_LOOP ( 'NONE', ( #23773, #43014 ) ) ;
#18514=DIRECTION ( 'NONE',  ( 0.000000000000000000, -1.000000000000000000, 0.000000000000000000 ) ) ;
#18522=DIRECTION ( 'NONE',  ( 1.000000000000000000, 0.000000000000000000, 0.000000000000000000 ) ) ;
#18536=ORIENTED_EDGE ( 'NONE', *, *, #5443, .T. ) ;
#18570=VECTOR ( 'NONE', #43437, 1000.000000000000000 ) ;
#18574=DIRECTION ( 'NONE',  ( 0.000000000000000000, -0.6438296778008192334, -0.7651688349527138167 ) ) ;
#18586=FACE_OUTER_BOUND ( 'NONE', #22176, .T. ) ;
#18601=CIRCLE ( 'NONE', #11247, 8.000000000000007105 ) ;
#18621=PLANE ( 'NONE',  #37829 ) ;
#18650=AXIS2_PLACEMENT_3D ( 'NONE', #24905, #38543, #35522 ) ;
#18668=FACE_OUTER_BOUND ( 'NONE', #44898, .T. ) ;
#18671=FACE_OUTER_BOUND ( 'NONE', #3243, .T. ) ;
#18714=AXIS2_PLACEMENT_3D ( 'NONE', #41792, #6453, #31147 ) ;
#18731=VECTOR ( 'NONE', #18111, 1000.000000000000000 ) ;
#18745=VECTOR ( 'NONE', #32711, 1000.000000000000000 ) ;
#18752=EDGE_CURVE ( 'NONE', #26579, #28289, #22746, .T. ) ;
#18803=CARTESIAN_POINT ( 'NONE',  ( 998.9999999999992042, 479.9999999999999432, -360.0000000000000000 ) ) ;
#18844=DIRECTION ( 'NONE',  ( 1.000000000000000000, 0.000000000000000000, 0.000000000000000000 ) ) ;
#18852=LINE ( 'NONE', #33161, #42949 ) ;
#18865=DIRECTION ( 'NONE',  ( -0.000000000000000000, -0.000000000000000000, 1.000000000000000000 ) ) ;
#18920=ORIENTED_EDGE ( 'NONE', *, *, #32349, .T. ) ;
#18976=CARTESIAN_POINT ( 'NONE',  ( 939.9999999999992042, 62.85347435602262323, 357.4246812887967621 ) ) ;
#19023=LINE ( 'NONE', #1451, #37923 ) ;
#19102=ORIENTED_EDGE ( 'NONE', *, *, #35641, .T. ) ;
#19126=EDGE_CURVE ( 'NONE', #25632, #30441, #30132, .T. ) ;
#19171=DIRECTION ( 'NONE',  ( 0.000000000000000000, -1.000000000000000000, 1.672022627447525240E-16 ) ) ;
#19176=VERTEX_POINT ( 'NONE', #45305 ) ;
#19267=LINE ( 'NONE', #33356, #7851 ) ;
#19314=ADVANCED_FACE ( 'NONE', ( #2244, #36904, #19575 ), #28904, .T. ) ;
#19327=CARTESIAN_POINT ( 'NONE',  ( 998.9999999999992042, -600.0000000000001137, 360.0000000000000000 ) ) ;
#19336=CARTESIAN_POINT ( 'NONE',  ( 914.9999999999992042, -426.1357934546398383, 350.0000000000000000 ) ) ;
#19385=ORIENTED_EDGE ( 'NONE', *, *, #28721, .T. ) ;
#19432=ORIENTED_EDGE ( 'NONE', *, *, #19626, .T. ) ;
#19451=DIRECTION ( 'NONE',  ( -0.000000000000000000, -0.000000000000000000, 1.000000000000000000 ) ) ;
#19468=ORIENTED_EDGE ( 'NONE', *, *, #19642, .T. ) ;
#19483=AXIS2_PLACEMENT_3D ( 'NONE', #7659, #22404, #39552 ) ;
#19493=EDGE_LOOP ( 'NONE', ( #6072, #16530, #35913, #5857 ) ) ;
#19575=FACE_OUTER_BOUND ( 'NONE', #7829, .T. ) ;
#19582=CARTESIAN_POINT ( 'NONE',  ( 919.9999999999993179, 154.9999999999998863, 350.0000000000000000 ) ) ;
#19585=ADVANCED_FACE ( 'NONE', ( #41059 ), #5939, .F. ) ;
#19598=ORIENTED_EDGE ( 'NONE', *, *, #12322, .F. ) ;
#19626=EDGE_CURVE ( 'NONE', #16198, #41554, #27197, .T. ) ;
#19642=EDGE_CURVE ( 'NONE', #11789, #14175, #20931, .T. ) ;
#19655=LINE ( 'NONE', #12717, #5726 ) ;
#19675=VECTOR ( 'NONE', #9850, 1000.000000000000000 ) ;
#19676=CARTESIAN_POINT ( 'NONE',  ( 989.9999999999992042, 249.9999999999998863, 360.0000000000000000 ) ) ;
#19680=FACE_BOUND ( 'NONE', #30172, .T. ) ;
#19682=EDGE_CURVE ( 'NONE', #23400, #16465, #12877, .T. ) ;
#19704=CARTESIAN_POINT ( 'NONE',  ( 914.9999999999992042, 99.99999999999984368, -360.0000000000000000 ) ) ;
#19714=CARTESIAN_POINT ( 'NONE',  ( 919.9999999999993179, 219.9999999999998863, 360.0000000000000000 ) ) ;
#19715=EDGE_LOOP ( 'NONE', ( #17871, #354, #25476, #38717 ) ) ;
#19787=DIRECTION ( 'NONE',  ( -0.000000000000000000, 0.000000000000000000, 1.000000000000000000 ) ) ;
#19829=ORIENTED_EDGE ( 'NONE', *, *, #3269, .T. ) ;
#19913=( NAMED_UNIT ( * ) PLANE_ANGLE_UNIT ( ) SI_UNIT ( $, .RADIAN. ) );
#19933=CARTESIAN_POINT ( 'NONE',  ( 989.9999999999992042, 50.81038600091411439, -210.0000000000000000 ) ) ;
#19942=ORIENTED_EDGE ( 'NONE', *, *, #31883, .T. ) ;
#19944=EDGE_CURVE ( 'NONE', #6307, #9644, #22079, .T. ) ;
#19956=EDGE_CURVE ( 'NONE', #26579, #30556, #28799, .T. ) ;
#20003=ORIENTED_EDGE ( 'NONE', *, *, #23281, .F. ) ;
#20038=DIRECTION ( 'NONE',  ( 0.000000000000000000, 0.000000000000000000, 1.000000000000000000 ) ) ;
#20045=EDGE_LOOP ( 'NONE', ( #10689, #23395, #7459, #36124 ) ) ;
#20070=ORIENTED_EDGE ( 'NONE', *, *, #11760, .F. ) ;
#20180=CYLINDRICAL_SURFACE ( 'NONE', #28428, 7.999999999999896083 ) ;
#20191=LINE ( 'NONE', #1951, #2407 ) ;
#20198=DIRECTION ( 'NONE',  ( 0.000000000000000000, 1.000000000000000000, -0.000000000000000000 ) ) ;
#20242=FACE_OUTER_BOUND ( 'NONE', #41423, .T. ) ;
#20248=ORIENTED_EDGE ( 'NONE', *, *, #33765, .F. ) ;
#20253=AXIS2_PLACEMENT_3D ( 'NONE', #37003, #19451, #2345 ) ;
#20282=VECTOR ( 'NONE', #44863, 1000.000000000000000 ) ;
#20292=AXIS2_PLACEMENT_3D ( 'NONE', #14675, #28519, #28269 ) ;
#20310=DIRECTION ( 'NONE',  ( 0.000000000000000000, 0.000000000000000000, 1.000000000000000000 ) ) ;
#20336=DIRECTION ( 'NONE',  ( -0.000000000000000000, -1.000000000000000000, 0.000000000000000000 ) ) ;
#20449=ORIENTED_EDGE ( 'NONE', *, *, #40670, .F. ) ;
#20456=VERTEX_POINT ( 'NONE', #9128 ) ;
#20464=VERTEX_POINT ( 'NONE', #39890 ) ;
#20482=PLANE ( 'NONE',  #33614 ) ;
#20485=LINE ( 'NONE', #7322, #42199 ) ;
#20509=CARTESIAN_POINT ( 'NONE',  ( 989.9999999999992042, 56.78581973499402835, -212.6378164459127049 ) ) ;
#20634=CARTESIAN_POINT ( 'NONE',  ( 879.9999999999992042, 99.99999999999984368, 360.0000000000000000 ) ) ;
#20663=VERTEX_POINT ( 'NONE', #23881 ) ;
#20714=PLANE ( 'NONE',  #359 ) ;
#20719=CARTESIAN_POINT ( 'NONE',  ( 919.9999999999993179, 154.9999999999998863, 360.0000000000000000 ) ) ;
#20723=EDGE_CURVE ( 'NONE', #9965, #31705, #2197, .T. ) ;
#20728=VERTEX_POINT ( 'NONE', #9595 ) ;
#20745=DIRECTION ( 'NONE',  ( 0.000000000000000000, 0.000000000000000000, 1.000000000000000000 ) ) ;
#20784=ORIENTED_EDGE ( 'NONE', *, *, #31927, .T. ) ;
#20795=CARTESIAN_POINT ( 'NONE',  ( 939.9999999999992042, 240.0000000000000568, -210.0000000000000000 ) ) ;
#20834=ORIENTED_EDGE ( 'NONE', *, *, #26387, .T. ) ;
#20855=LINE ( 'NONE', #17653, #35159 ) ;
#20859=CARTESIAN_POINT ( 'NONE',  ( 989.9999999999992042, 62.85347435602256638, 357.4246812887967053 ) ) ;
#20918=DIRECTION ( 'NONE',  ( -0.000000000000000000, -0.000000000000000000, 1.000000000000000000 ) ) ;
#20931=LINE ( 'NONE', #41290, #13425 ) ;
#20941=CARTESIAN_POINT ( 'NONE',  ( 939.9999999999993179, -431.4567479753240491, 350.0000000000000000 ) ) ;
#20948=EDGE_LOOP ( 'NONE', ( #2055, #2742, #20070, #13024 ) ) ;
#21048=EDGE_CURVE ( 'NONE', #17397, #23953, #15850, .T. ) ;
#21049=AXIS2_PLACEMENT_3D ( 'NONE', #28084, #20918, #10089 ) ;
#21086=AXIS2_PLACEMENT_3D ( 'NONE', #3999, #24784, #32181 ) ;
#21100=LINE ( 'NONE', #14869, #2653 ) ;
#21132=CARTESIAN_POINT ( 'NONE',  ( 939.9999999999992042, 50.81038600091411439, -217.3872392842761769 ) ) ;
#21142=ORIENTED_EDGE ( 'NONE', *, *, #44180, .T. ) ;
#21182=CARTESIAN_POINT ( 'NONE',  ( 919.9999999999993179, 154.9999999999998863, -360.0000000000000000 ) ) ;
#21293=LINE ( 'NONE', #273, #45389 ) ;
#21305=EDGE_CURVE ( 'NONE', #17231, #13352, #39839, .T. ) ;
#21330=DIRECTION ( 'NONE',  ( 0.000000000000000000, 1.000000000000000000, -0.000000000000000000 ) ) ;
#21395=CARTESIAN_POINT ( 'NONE',  ( 914.9999999999992042, 99.99999999999984368, 360.0000000000000000 ) ) ;
#21420=DIRECTION ( 'NONE',  ( 1.000000000000000000, 0.000000000000000000, 0.000000000000000000 ) ) ;
#21446=CARTESIAN_POINT ( 'NONE',  ( 939.9999999999993179, -179.7356316342496712, 69.11609595480024382 ) ) ;
#21487=ORIENTED_EDGE ( 'NONE', *, *, #18752, .F. ) ;
#21514=CARTESIAN_POINT ( 'NONE',  ( 939.9999999999994316, -434.4637272565419153, 347.3621835540871530 ) ) ;
#21571=EDGE_CURVE ( 'NONE', #45702, #27431, #8911, .T. ) ;
#21581=ORIENTED_EDGE ( 'NONE', *, *, #7658, .F. ) ;
#21584=VECTOR ( 'NONE', #1224, 1000.000000000000000 ) ;
#21586=CARTESIAN_POINT ( 'NONE',  ( 989.9999999999992042, 249.9999999999998863, -209.9999999999999716 ) ) ;
#21609=DIRECTION ( 'NONE',  ( 0.000000000000000000, 0.000000000000000000, -1.000000000000000000 ) ) ;
#21614=DIRECTION ( 'NONE',  ( 0.000000000000000000, -0.6438296778008192334, -0.7651688349527138167 ) ) ;
#21637=CARTESIAN_POINT ( 'NONE',  ( 911.9749999999993406, 154.9999999999998863, 360.0000000000000000 ) ) ;
#21646=AXIS2_PLACEMENT_3D ( 'NONE', #34388, #13380, #44801 ) ;
#21647=ORIENTED_EDGE ( 'NONE', *, *, #23279, .T. ) ;
#21666=CARTESIAN_POINT ( 'NONE',  ( 989.9999999999992042, -426.1357934546398383, 350.0000000000000000 ) ) ;
#21703=DIRECTION ( 'NONE',  ( 1.000000000000000000, 0.000000000000000000, 0.000000000000000000 ) ) ;
#21754=ORIENTED_EDGE ( 'NONE', *, *, #13193, .F. ) ;
#21787=AXIS2_PLACEMENT_3D ( 'NONE', #12386, #33849, #22536 ) ;
#21808=DIRECTION ( 'NONE',  ( -4.625929269271485914E-16, 1.000000000000000000, 0.000000000000000000 ) ) ;
#21812=CIRCLE ( 'NONE', #40261, 8.024999999999948841 ) ;
#21851=VECTOR ( 'NONE', #21609, 1000.000000000000000 ) ;
#21874=ORIENTED_EDGE ( 'NONE', *, *, #8301, .F. ) ;
#21881=ORIENTED_EDGE ( 'NONE', *, *, #27795, .T. ) ;
#21882=VECTOR ( 'NONE', #31828, 1000.000000000000114 ) ;
#21883=EDGE_CURVE ( 'NONE', #39622, #15578, #29927, .T. ) ;
#21893=ORIENTED_EDGE ( 'NONE', *, *, #4624, .F. ) ;
#21898=AXIS2_PLACEMENT_3D ( 'NONE', #31092, #6398, #45191 ) ;
#21978=CARTESIAN_POINT ( 'NONE',  ( 999.9999999999992042, 239.9999999999998863, 360.0000000000000000 ) ) ;
#22039=CARTESIAN_POINT ( 'NONE',  ( 989.9999999999992042, 249.9999999999998863, 360.0000000000000000 ) ) ;
#22043=ORIENTED_EDGE ( 'NONE', *, *, #40217, .T. ) ;
#22079=CIRCLE ( 'NONE', #4029, 7.999999999999785061 ) ;
#22144=DIRECTION ( 'NONE',  ( -0.000000000000000000, -0.000000000000000000, -1.000000000000000000 ) ) ;
#22159=EDGE_CURVE ( 'NONE', #23669, #37975, #27594, .T. ) ;
#22160=EDGE_LOOP ( 'NONE', ( #15573, #36687, #1354, #8308 ) ) ;
#22176=EDGE_LOOP ( 'NONE', ( #4407, #40305, #37332, #26136 ) ) ;
#22237=FACE_BOUND ( 'NONE', #3321, .T. ) ;
#22334=CARTESIAN_POINT ( 'NONE',  ( 989.9999999999992042, 469.9999999999999432, -210.0000000000000000 ) ) ;
#22335=CARTESIAN_POINT ( 'NONE',  ( 939.9999999999992042, 62.85347435602262323, 357.4246812887967621 ) ) ;
#22339=ADVANCED_FACE ( 'NONE', ( #2664 ), #13294, .T. ) ;
#22365=VECTOR ( 'NONE', #26913, 1000.000000000000000 ) ;
#22398=CARTESIAN_POINT ( 'NONE',  ( 989.9999999999992042, -414.5899773927342835, -209.9999999999999716 ) ) ;
#22404=DIRECTION ( 'NONE',  ( -0.000000000000000000, -0.000000000000000000, -1.000000000000000000 ) ) ;
#22430=VERTEX_POINT ( 'NONE', #18133 ) ;
#22434=ADVANCED_FACE ( 'NONE', ( #11418 ), #28975, .F. ) ;
#22454=AXIS2_PLACEMENT_3D ( 'NONE', #29133, #8129, #32599 ) ;
#22456=CARTESIAN_POINT ( 'NONE',  ( 187.1337867209877857, -185.0721577059061644, 75.19946970736494052 ) ) ;
#22536=DIRECTION ( 'NONE',  ( 0.000000000000000000, -0.6594541114781790059, 0.7517448203044204691 ) ) ;
#22539=VECTOR ( 'NONE', #45182, 1000.000000000000000 ) ;
#22562=LINE ( 'NONE', #19327, #31400 ) ;
#22619=CARTESIAN_POINT ( 'NONE',  ( 928.0249999999991815, 219.9999999999998863, 360.0000000000000000 ) ) ;
#22627=ORIENTED_EDGE ( 'NONE', *, *, #4735, .F. ) ;
#22728=EDGE_CURVE ( 'NONE', #28192, #11754, #9074, .T. ) ;
#22746=LINE ( 'NONE', #43325, #27656 ) ;
#22769=CARTESIAN_POINT ( 'NONE',  ( 879.9999999999992042, 249.9999999999998295, -199.9999999999997442 ) ) ;
#22791=FACE_OUTER_BOUND ( 'NONE', #32794, .T. ) ;
#22875=FACE_OUTER_BOUND ( 'NONE', #14171, .T. ) ;
#22944=FACE_OUTER_BOUND ( 'NONE', #15272, .T. ) ;
#22959=CARTESIAN_POINT ( 'NONE',  ( 939.9999999999993179, -600.0000000000001137, 350.0000000000000000 ) ) ;
#23110=ORIENTED_EDGE ( 'NONE', *, *, #25847, .T. ) ;
#23117=ORIENTED_EDGE ( 'NONE', *, *, #30060, .T. ) ;
#23119=FACE_BOUND ( 'NONE', #5176, .T. ) ;
#23134=DIRECTION ( 'NONE',  ( 1.000000000000000000, -0.000000000000000000, -0.000000000000000000 ) ) ;
#23140=VECTOR ( 'NONE', #34958, 1000.000000000000114 ) ;
#23148=CARTESIAN_POINT ( 'NONE',  ( 914.9999999999992042, 74.99999999999984368, 350.0000000000000000 ) ) ;
#23153=CARTESIAN_POINT ( 'NONE',  ( 0.000000000000000000, 0.000000000000000000, 0.000000000000000000 ) ) ;
#23159=AXIS2_PLACEMENT_3D ( 'NONE', #16004, #26606, #30774 ) ;
#23165=LINE ( 'NONE', #33815, #1184 ) ;
#23181=DIRECTION ( 'NONE',  ( 0.000000000000000000, 1.000000000000000000, -0.000000000000000000 ) ) ;
#23210=CARTESIAN_POINT ( 'NONE',  ( 999.9999999999992042, 249.9999999999998863, 360.0000000000000000 ) ) ;
#23232=DIRECTION ( 'NONE',  ( 1.000000000000000000, 0.000000000000000000, 0.000000000000000000 ) ) ;
#23255=AXIS2_PLACEMENT_3D ( 'NONE', #25732, #21808, #11419 ) ;
#23271=EDGE_CURVE ( 'NONE', #41554, #44486, #44962, .T. ) ;
#23276=ORIENTED_EDGE ( 'NONE', *, *, #35704, .T. ) ;
#23279=EDGE_CURVE ( 'NONE', #19176, #22430, #3381, .T. ) ;
#23281=EDGE_CURVE ( 'NONE', #861, #14052, #27394, .T. ) ;
#23318=CARTESIAN_POINT ( 'NONE',  ( 989.9999999999992042, -434.4637272565419153, 347.3621835540870393 ) ) ;
#23359=LINE ( 'NONE', #44619, #26320 ) ;
#23395=ORIENTED_EDGE ( 'NONE', *, *, #2079, .T. ) ;
#23400=VERTEX_POINT ( 'NONE', #13783 ) ;
#23407=CARTESIAN_POINT ( 'NONE',  ( 927.9999999999990905, 154.9999999999998863, -360.0000000000000000 ) ) ;
#23408=CARTESIAN_POINT ( 'NONE',  ( 999.9999999999992042, 249.9999999999998863, 360.0000000000000000 ) ) ;
#23442=ORIENTED_EDGE ( 'NONE', *, *, #31181, .T. ) ;
#23458=EDGE_LOOP ( 'NONE', ( #35670, #1680, #28111 ) ) ;
#23464=LINE ( 'NONE', #5237, #12940 ) ;
#23487=ORIENTED_EDGE ( 'NONE', *, *, #8323, .F. ) ;
#23501=ORIENTED_EDGE ( 'NONE', *, *, #33439, .F. ) ;
#23619=VERTEX_POINT ( 'NONE', #35459 ) ;
#23669=VERTEX_POINT ( 'NONE', #28775 ) ;
#23705=DIRECTION ( 'NONE',  ( 0.000000000000000000, 0.7517448203044204691, 0.6594541114781790059 ) ) ;
#23732=EDGE_CURVE ( 'NONE', #34939, #8196, #39643, .T. ) ;
#23742=DIRECTION ( 'NONE',  ( 0.000000000000000000, 0.000000000000000000, -1.000000000000000000 ) ) ;
#23773=ORIENTED_EDGE ( 'NONE', *, *, #42141, .F. ) ;
#23802=ORIENTED_EDGE ( 'NONE', *, *, #25847, .F. ) ;
#23821=AXIS2_PLACEMENT_3D ( 'NONE', #44981, #155, #35256 ) ;
#23830=ORIENTED_EDGE ( 'NONE', *, *, #32349, .F. ) ;
#23836=DIRECTION ( 'NONE',  ( -1.000000000000000000, 0.000000000000000000, 0.000000000000000000 ) ) ;
#23837=EDGE_LOOP ( 'NONE', ( #5805, #30341, #26034, #21581 ) ) ;
#23862=LINE ( 'NONE', #20859, #23140 ) ;
#23873=CARTESIAN_POINT ( 'NONE',  ( 998.9999999999992042, -599.0000000000001137, 360.0000000000000000 ) ) ;
#23881=CARTESIAN_POINT ( 'NONE',  ( 989.9999999999992042, -419.8175818341089780, -209.9999999999999716 ) ) ;
#23886=ADVANCED_FACE ( 'NONE', ( #22944 ), #30121, .F. ) ;
#23887=FACE_OUTER_BOUND ( 'NONE', #31341, .T. ) ;
#23953=VERTEX_POINT ( 'NONE', #29666 ) ;
#23959=ORIENTED_EDGE ( 'NONE', *, *, #19682, .T. ) ;
#23976=CYLINDRICAL_SURFACE ( 'NONE', #18714, 7.999999999999896083 ) ;
#24008=ORIENTED_EDGE ( 'NONE', *, *, #10551, .T. ) ;
#24065=ORIENTED_EDGE ( 'NONE', *, *, #25793, .F. ) ;
#24092=DIRECTION ( 'NONE',  ( 0.000000000000000000, 0.000000000000000000, 1.000000000000000000 ) ) ;
#24112=CARTESIAN_POINT ( 'NONE',  ( 999.9999999999992042, -590.0000000000001137, 360.0000000000000000 ) ) ;
#24136=EDGE_CURVE ( 'NONE', #36984, #34629, #23165, .T. ) ;
#24199=ORIENTED_EDGE ( 'NONE', *, *, #43343, .T. ) ;
#24216=CYLINDRICAL_SURFACE ( 'NONE', #4932, 24.99999999999991118 ) ;
#24231=CARTESIAN_POINT ( 'NONE',  ( 999.9999999999992042, 478.9999999999999432, -359.0000000000000000 ) ) ;
#24273=AXIS2_PLACEMENT_3D ( 'NONE', #27937, #10379, #24455 ) ;
#24314=ADVANCED_FACE ( 'NONE', ( #6087 ), #35566, .T. ) ;
#24338=PLANE ( 'NONE',  #13569 ) ;
#24350=DIRECTION ( 'NONE',  ( -0.000000000000000000, -0.000000000000000000, 1.000000000000000000 ) ) ;
#24398=EDGE_CURVE ( 'NONE', #20663, #29615, #32805, .T. ) ;
#24400=VERTEX_POINT ( 'NONE', #22619 ) ;
#24438=CYLINDRICAL_SURFACE ( 'NONE', #18650, 24.99999999999991118 ) ;
#24455=DIRECTION ( 'NONE',  ( 1.000000000000000000, 0.000000000000000000, 0.000000000000000000 ) ) ;
#24542=ORIENTED_EDGE ( 'NONE', *, *, #11724, .T. ) ;
#24558=CARTESIAN_POINT ( 'NONE',  ( 187.1337867209877857, 62.85347435602256638, 357.4246812887967053 ) ) ;
#24572=CARTESIAN_POINT ( 'NONE',  ( 911.9999999999993179, 154.9999999999998863, 360.0000000000000000 ) ) ;
#24580=DIRECTION ( 'NONE',  ( -1.084653538143406060E-16, 0.6594541114781790059, -0.7517448203044204691 ) ) ;
#24606=DIRECTION ( 'NONE',  ( 0.000000000000000000, -0.7651688349527138167, 0.6438296778008192334 ) ) ;
#24624=AXIS2_PLACEMENT_3D ( 'NONE', #24112, #20198, #27143 ) ;
#24657=ADVANCED_FACE ( 'NONE', ( #5079 ), #26080, .T. ) ;
#24719=VERTEX_POINT ( 'NONE', #12462 ) ;
#24721=DIRECTION ( 'NONE',  ( 1.000000000000000000, 0.000000000000000000, 0.000000000000000000 ) ) ;
#24751=VECTOR ( 'NONE', #16553, 1000.000000000000000 ) ;
#24784=DIRECTION ( 'NONE',  ( -1.000000000000000000, 0.000000000000000000, 0.000000000000000000 ) ) ;
#24789=CARTESIAN_POINT ( 'NONE',  ( 939.9999999999993179, -590.0000000000001137, 360.0000000000000000 ) ) ;
#24835=AXIS2_PLACEMENT_3D ( 'NONE', #19676, #34202, #9736 ) ;
#24843=ORIENTED_EDGE ( 'NONE', *, *, #6551, .F. ) ;
#24849=FACE_OUTER_BOUND ( 'NONE', #39629, .T. ) ;
#24904=DIRECTION ( 'NONE',  ( 1.000000000000000000, 0.000000000000000000, -0.000000000000000000 ) ) ;
#24905=CARTESIAN_POINT ( 'NONE',  ( 914.9999999999992042, 74.99999999999984368, 360.0000000000000000 ) ) ;
#24937=DIRECTION ( 'NONE',  ( 1.000000000000000000, 1.644774851296528363E-16, -0.000000000000000000 ) ) ;
#25016=FACE_OUTER_BOUND ( 'NONE', #4459, .T. ) ;
#25020=DIRECTION ( 'NONE',  ( -0.000000000000000000, -0.000000000000000000, 1.000000000000000000 ) ) ;
#25032=DIRECTION ( 'NONE',  ( 1.000000000000000000, -0.000000000000000000, 0.000000000000000000 ) ) ;
#25045=DIRECTION ( 'NONE',  ( -0.000000000000000000, -0.000000000000000000, 1.000000000000000000 ) ) ;
#25071=CARTESIAN_POINT ( 'NONE',  ( 998.9999999999992042, 249.9999999999998863, 360.0000000000000000 ) ) ;
#25091=CARTESIAN_POINT ( 'NONE',  ( 939.9999999999993179, 56.78581973499407809, -212.6378164459127618 ) ) ;
#25110=ORIENTED_EDGE ( 'NONE', *, *, #35912, .T. ) ;
#25135=CARTESIAN_POINT ( 'NONE',  ( 999.9999999999992042, -600.0000000000001137, -360.0000000000000000 ) ) ;
#25161=CARTESIAN_POINT ( 'NONE',  ( 939.9999999999993179, -600.0000000000001137, 360.0000000000000000 ) ) ;
#25163=ORIENTED_EDGE ( 'NONE', *, *, #14227, .T. ) ;
#25178=ORIENTED_EDGE ( 'NONE', *, *, #9772, .F. ) ;
#25185=LINE ( 'NONE', #7207, #6781 ) ;
#25201=STYLED_ITEM('',(#45744),#17219);
#25208=ORIENTED_EDGE ( 'NONE', *, *, #39964, .T. ) ;
#25218=ORIENTED_EDGE ( 'NONE', *, *, #19956, .F. ) ;
#25235=CARTESIAN_POINT ( 'NONE',  ( 989.9999999999992042, 56.73212367640085318, 362.5753187112032379 ) ) ;
#25266=CARTESIAN_POINT ( 'NONE',  ( 919.9999999999993179, 154.9999999999998863, 359.9749999999999659 ) ) ;
#25270=EDGE_CURVE ( 'NONE', #20663, #4785, #31611, .T. ) ;
#25294=ORIENTED_EDGE ( 'NONE', *, *, #11400, .T. ) ;
#25313=EDGE_CURVE ( 'NONE', #38247, #12844, #28138, .T. ) ;
#25318=DIRECTION ( 'NONE',  ( -0.000000000000000000, -0.000000000000000000, -1.000000000000000000 ) ) ;
#25375=LINE ( 'NONE', #4376, #29911 ) ;
#25394=DIRECTION ( 'NONE',  ( 1.000000000000000000, -0.000000000000000000, -0.000000000000000000 ) ) ;
#25415=ORIENTED_EDGE ( 'NONE', *, *, #33439, .T. ) ;
#25433=DIRECTION ( 'NONE',  ( -1.058954862565134068E-16, 0.6438296778008191223, 0.7651688349527137056 ) ) ;
#25476=ORIENTED_EDGE ( 'NONE', *, *, #28401, .F. ) ;
#25481=CARTESIAN_POINT ( 'NONE',  ( 939.9999999999992042, 46.15097736693707020, 350.0000000000000000 ) ) ;
#25489=FACE_OUTER_BOUND ( 'NONE', #7466, .T. ) ;
#25499=ORIENTED_EDGE ( 'NONE', *, *, #25793, .T. ) ;
#25517=AXIS2_PLACEMENT_3D ( 'NONE', #1678, #15782, #40507 ) ;
#25562=ADVANCED_FACE ( 'NONE', ( #18668 ), #8269, .T. ) ;
#25581=ORIENTED_EDGE ( 'NONE', *, *, #19642, .F. ) ;
#25587=EDGE_CURVE ( 'NONE', #34011, #23619, #11280, .T. ) ;
#25597=CARTESIAN_POINT ( 'NONE',  ( 989.9999999999992042, 56.78581973499402835, -212.6378164459127049 ) ) ;
#25606=LINE ( 'NONE', #29310, #37058 ) ;
#25615=VECTOR ( 'NONE', #39929, 1000.000000000000000 ) ;
#25619=AXIS2_PLACEMENT_3D ( 'NONE', #13249, #6306, #23836 ) ;
#25632=VERTEX_POINT ( 'NONE', #22334 ) ;
#25639=( BOUNDED_CURVE ( )  B_SPLINE_CURVE ( 3, ( #34819, #16602, #3424, #30685 ),
 .UNSPECIFIED., .F., .T. ) 
 B_SPLINE_CURVE_WITH_KNOTS ( ( 4, 4 ),
 ( 3.141592653589793116, 4.712388980384689674 ),
 .UNSPECIFIED. ) 
 CURVE ( )  GEOMETRIC_REPRESENTATION_ITEM ( )  RATIONAL_B_SPLINE_CURVE ( ( 1.000000000000000000, 0.8047378541243649375, 0.8047378541243649375, 1.000000000000000000 ) ) 
 REPRESENTATION_ITEM ( '' )  );
#25647=VERTEX_POINT ( 'NONE', #21666 ) ;
#25732=CARTESIAN_POINT ( 'NONE',  ( -2.174186756557595869E-13, 469.9999999999994884, 0.000000000000000000 ) ) ;
#25751=ORIENTED_EDGE ( 'NONE', *, *, #12005, .T. ) ;
#25764=DIRECTION ( 'NONE',  ( 1.000000000000000000, 0.000000000000000000, 0.000000000000000000 ) ) ;
#25793=EDGE_CURVE ( 'NONE', #11392, #37728, #35995, .T. ) ;
#25815=EDGE_CURVE ( 'NONE', #28192, #20456, #8502, .T. ) ;
#25817=CARTESIAN_POINT ( 'NONE',  ( 989.9999999999992042, 249.9999999999998863, 360.0000000000000000 ) ) ;
#25847=EDGE_CURVE ( 'NONE', #11392, #42107, #1729, .T. ) ;
#25864=CARTESIAN_POINT ( 'NONE',  ( 939.9999999999993179, -600.0000000000001137, 360.0000000000000000 ) ) ;
#25867=ORIENTED_EDGE ( 'NONE', *, *, #16989, .T. ) ;
#25922=FACE_BOUND ( 'NONE', #23458, .T. ) ;
#25924=CARTESIAN_POINT ( 'NONE',  ( 939.9999999999992042, 74.99999999999984368, 360.0000000000000000 ) ) ;
#25928=DIRECTION ( 'NONE',  ( 0.000000000000000000, 0.000000000000000000, 1.000000000000000000 ) ) ;
#25938=VERTEX_POINT ( 'NONE', #26710 ) ;
#25949=PLANE ( 'NONE',  #2766 ) ;
#25965=DIRECTION ( 'NONE',  ( 0.000000000000000000, 1.000000000000000000, -0.000000000000000000 ) ) ;
#25978=CARTESIAN_POINT ( 'NONE',  ( 998.9999999999992042, 249.9999999999998863, 360.0000000000000000 ) ) ;
#26011=ORIENTED_EDGE ( 'NONE', *, *, #27506, .F. ) ;
#26034=ORIENTED_EDGE ( 'NONE', *, *, #13086, .T. ) ;
#26080=PLANE ( 'NONE',  #3430 ) ;
#26136=ORIENTED_EDGE ( 'NONE', *, *, #15654, .F. ) ;
#26147=EDGE_CURVE ( 'NONE', #20728, #41166, #30185, .T. ) ;
#26157=CARTESIAN_POINT ( 'NONE',  ( 998.9999999999992042, 479.9999999999999432, -199.9999999999999716 ) ) ;
#26160=DIRECTION ( 'NONE',  ( -1.000000000000000000, -4.625929269271485914E-16, 0.000000000000000000 ) ) ;
#26166=VECTOR ( 'NONE', #45212, 1000.000000000000000 ) ;
#26177=DIRECTION ( 'NONE',  ( 1.000000000000000000, 0.000000000000000000, 0.000000000000000000 ) ) ;
#26197=ORIENTED_EDGE ( 'NONE', *, *, #36847, .F. ) ;
#26208=DIRECTION ( 'NONE',  ( -0.000000000000000000, -0.6438296778008192334, -0.7651688349527135946 ) ) ;
#26230=VECTOR ( 'NONE', #42647, 1000.000000000000000 ) ;
#26268=VECTOR ( 'NONE', #31121, 1000.000000000000000 ) ;
#26289=LINE ( 'NONE', #15895, #38709 ) ;
#26298=ORIENTED_EDGE ( 'NONE', *, *, #693, .T. ) ;
#26306=ORIENTED_EDGE ( 'NONE', *, *, #12906, .F. ) ;
#26307=ORIENTED_EDGE ( 'NONE', *, *, #26147, .T. ) ;
#26320=VECTOR ( 'NONE', #37460, 1000.000000000000000 ) ;
#26359=DIRECTION ( 'NONE',  ( 0.000000000000000000, 0.000000000000000000, 1.000000000000000000 ) ) ;
#26380=PLANE ( 'NONE',  #24835 ) ;
#26385=CARTESIAN_POINT ( 'NONE',  ( 879.9999999999992042, 99.99999999999984368, 360.0000000000000000 ) ) ;
#26387=EDGE_CURVE ( 'NONE', #14052, #33479, #35013, .T. ) ;
#26391=LINE ( 'NONE', #36568, #42489 ) ;
#26409=ADVANCED_FACE ( 'NONE', ( #20242 ), #38123, .F. ) ;
#26417=ORIENTED_EDGE ( 'NONE', *, *, #14833, .T. ) ;
#26420=EDGE_CURVE ( 'NONE', #17231, #16198, #9444, .T. ) ;
#26426=VECTOR ( 'NONE', #7556, 1000.000000000000000 ) ;
#26445=DIRECTION ( 'NONE',  ( 0.000000000000000000, 0.000000000000000000, 1.000000000000000000 ) ) ;
#26451=CARTESIAN_POINT ( 'NONE',  ( 989.9999999999992042, 62.85347435602256638, 357.4246812887967053 ) ) ;
#26461=DIRECTION ( 'NONE',  ( -0.000000000000000000, -0.000000000000000000, -1.000000000000000000 ) ) ;
#26464=FACE_OUTER_BOUND ( 'NONE', #45343, .T. ) ;
#26473=ORIENTED_EDGE ( 'NONE', *, *, #30371, .F. ) ;
#26516=ADVANCED_FACE ( 'NONE', ( #45430 ), #31773, .T. ) ;
#26526=CARTESIAN_POINT ( 'NONE',  ( 187.1337867209877857, -184.9457194955397199, 62.92409052808242365 ) ) ;
#26527=ORIENTED_EDGE ( 'NONE', *, *, #33765, .T. ) ;
#26546=ORIENTED_EDGE ( 'NONE', *, *, #21883, .T. ) ;
#26576=ORIENTED_EDGE ( 'NONE', *, *, #30897, .T. ) ;
#26579=VERTEX_POINT ( 'NONE', #41735 ) ;
#26584=EDGE_LOOP ( 'NONE', ( #14633, #36708, #23802, #43980 ) ) ;
#26606=DIRECTION ( 'NONE',  ( -0.000000000000000000, -0.000000000000000000, -1.000000000000000000 ) ) ;
#26658=DIRECTION ( 'NONE',  ( 0.000000000000000000, 1.000000000000000000, -0.000000000000000000 ) ) ;
#26673=ADVANCED_FACE ( 'NONE', ( #24849 ), #14925, .F. ) ;
#26683=EDGE_LOOP ( 'NONE', ( #6207, #24843, #3995, #35612 ) ) ;
#26687=AXIS2_PLACEMENT_3D ( 'NONE', #11584, #18514, #42534 ) ;
#26704=DIRECTION ( 'NONE',  ( -0.000000000000000000, -0.000000000000000000, 1.000000000000000000 ) ) ;
#26710=CARTESIAN_POINT ( 'NONE',  ( 879.9999999999992042, 99.99999999999984368, -360.0000000000000000 ) ) ;
#26797=DIRECTION ( 'NONE',  ( -1.084653538143406060E-16, 0.6594541114781790059, -0.7517448203044204691 ) ) ;
#26800=AXIS2_PLACEMENT_3D ( 'NONE', #4623, #11795, #15269 ) ;
#26802=ORIENTED_EDGE ( 'NONE', *, *, #11170, .T. ) ;
#26813=AXIS2_PLACEMENT_3D ( 'NONE', #25161, #24937, #36473 ) ;
#26840=CARTESIAN_POINT ( 'NONE',  ( 187.1337867209877857, 50.81038600091411439, -193.6948738798775764 ) ) ;
#26841=DIRECTION ( 'NONE',  ( 0.000000000000000000, 0.000000000000000000, -1.000000000000000000 ) ) ;
#26844=ORIENTED_EDGE ( 'NONE', *, *, #28896, .T. ) ;
#26850=FACE_OUTER_BOUND ( 'NONE', #12770, .T. ) ;
#26851=ORIENTED_EDGE ( 'NONE', *, *, #1846, .F. ) ;
#26858=AXIS2_PLACEMENT_3D ( 'NONE', #23153, #34241, #6075 ) ;
#26913=DIRECTION ( 'NONE',  ( -1.000000000000000000, -4.625929269271485914E-16, 0.000000000000000000 ) ) ;
#26926=ORIENTED_EDGE ( 'NONE', *, *, #40756, .T. ) ;
#26962=CARTESIAN_POINT ( 'NONE',  ( 1820.038553321469863, 47.45399382421944523, -201.9999999999999432 ) ) ;
#26987=LINE ( 'NONE', #30220, #9190 ) ;
#26989=EDGE_LOOP ( 'NONE', ( #25581, #41755, #33144, #32123 ) ) ;
#27024=CARTESIAN_POINT ( 'NONE',  ( 989.9999999999992042, -407.8586036264140375, -201.9999999999998863 ) ) ;
#27040=ORIENTED_EDGE ( 'NONE', *, *, #10062, .T. ) ;
#27125=CARTESIAN_POINT ( 'NONE',  ( 989.9999999999992042, 62.85347435602256638, 357.4246812887967053 ) ) ;
#27134=CARTESIAN_POINT ( 'NONE',  ( 999.9999999999992042, 478.9999999999999432, -200.9999999999999432 ) ) ;
#27143=DIRECTION ( 'NONE',  ( 0.000000000000000000, 0.000000000000000000, 1.000000000000000000 ) ) ;
#27192=DIRECTION ( 'NONE',  ( 0.000000000000000000, 0.000000000000000000, -1.000000000000000000 ) ) ;
#27197=LINE ( 'NONE', #10323, #36265 ) ;
#27265=ADVANCED_FACE ( 'NONE', ( #40987 ), #5401, .F. ) ;
#27345=FACE_OUTER_BOUND ( 'NONE', #40251, .T. ) ;
#27349=PLANE ( 'NONE',  #291 ) ;
#27374=ORIENTED_EDGE ( 'NONE', *, *, #38685, .F. ) ;
#27379=CARTESIAN_POINT ( 'NONE',  ( 989.9999999999992042, -190.2822455671962416, 69.00746428064729798 ) ) ;
#27394=LINE ( 'NONE', #31314, #22539 ) ;
#27402=CARTESIAN_POINT ( 'NONE',  ( 999.5857864376259840, 479.9999999999999432, -199.9999999999999432 ) ) ;
#27431=VERTEX_POINT ( 'NONE', #10250 ) ;
#27453=FACE_OUTER_BOUND ( 'NONE', #28465, .T. ) ;
#27472=ADVANCED_FACE ( 'NONE', ( #17180 ), #27349, .T. ) ;
#27506=EDGE_CURVE ( 'NONE', #33095, #20456, #23862, .T. ) ;
#27533=CIRCLE ( 'NONE', #26800, 8.024999999999948841 ) ;
#27545=ORIENTED_EDGE ( 'NONE', *, *, #37043, .F. ) ;
#27549=EDGE_LOOP ( 'NONE', ( #1975, #44306, #29329, #14790 ) ) ;
#27567=ORIENTED_EDGE ( 'NONE', *, *, #32926, .F. ) ;
#27594=LINE ( 'NONE', #31739, #17376 ) ;
#27626=CARTESIAN_POINT ( 'NONE',  ( 999.9999999999992042, 479.5857864376268935, -200.4142135623730496 ) ) ;
#27635=CONICAL_SURFACE ( 'NONE', #3311, 8.024999999999948841, 0.7853981633963380560 ) ;
#27652=CARTESIAN_POINT ( 'NONE',  ( 939.9999999999993179, -600.0000000000001137, -350.0000000000000000 ) ) ;
#27656=VECTOR ( 'NONE', #36165, 1000.000000000000000 ) ;
#27661=ORIENTED_EDGE ( 'NONE', *, *, #14227, .F. ) ;
#27670=ADVANCED_BREP_SHAPE_REPRESENTATION ( '', ( #17219, #26858 ), #39435 ) ;
#27702=DIRECTION ( 'NONE',  ( 1.644774851296528363E-16, -1.000000000000000000, 0.000000000000000000 ) ) ;
#27709=CARTESIAN_POINT ( 'NONE',  ( 939.9999999999993179, -407.8586036264139807, -201.9999999999998863 ) ) ;
#27763=EDGE_CURVE ( 'NONE', #29887, #8835, #35637, .T. ) ;
#27764=CARTESIAN_POINT ( 'NONE',  ( 187.1337867209877857, 62.85347435602256638, 357.4246812887967053 ) ) ;
#27795=EDGE_CURVE ( 'NONE', #1032, #42107, #4257, .T. ) ;
#27804=LINE ( 'NONE', #10468, #40997 ) ;
#27892=DIRECTION ( 'NONE',  ( 1.000000000000000000, 4.625929269271485914E-16, 0.000000000000000000 ) ) ;
#27897=DIRECTION ( 'NONE',  ( 1.000000000000000000, 0.000000000000000000, 0.000000000000000000 ) ) ;
#27904=VERTEX_POINT ( 'NONE', #25481 ) ;
#27937=CARTESIAN_POINT ( 'NONE',  ( 919.9999999999993179, 219.9999999999998863, 350.0000000000000000 ) ) ;
#27988=FACE_OUTER_BOUND ( 'NONE', #33809, .T. ) ;
#28037=CARTESIAN_POINT ( 'NONE',  ( 939.9999999999992042, 74.99999999999984368, 360.0000000000000000 ) ) ;
#28052=LINE ( 'NONE', #21132, #7793 ) ;
#28084=CARTESIAN_POINT ( 'NONE',  ( 919.9999999999993179, 219.9999999999998863, 360.0000000000000000 ) ) ;
#28111=ORIENTED_EDGE ( 'NONE', *, *, #37641, .F. ) ;
#28113=VECTOR ( 'NONE', #15097, 1000.000000000000000 ) ;
#28115=DIRECTION ( 'NONE',  ( 0.000000000000000000, -0.6594541114781790059, 0.7517448203044204691 ) ) ;
#28122=EDGE_LOOP ( 'NONE', ( #20449, #37027 ) ) ;
#28138=LINE ( 'NONE', #17067, #33690 ) ;
#28141=DIRECTION ( 'NONE',  ( -1.000000000000000000, 0.000000000000000000, 0.000000000000000000 ) ) ;
#28192=VERTEX_POINT ( 'NONE', #8386 ) ;
#28228=VERTEX_POINT ( 'NONE', #29624 ) ;
#28269=DIRECTION ( 'NONE',  ( 1.000000000000000000, 0.000000000000000000, 0.000000000000000000 ) ) ;
#28285=EDGE_CURVE ( 'NONE', #14449, #15624, #43483, .T. ) ;
#28289=VERTEX_POINT ( 'NONE', #26385 ) ;
#28313=DIRECTION ( 'NONE',  ( -0.000000000000000000, -0.7517448203044211352, -0.6594541114781783397 ) ) ;
#28338=ADVANCED_FACE ( 'NONE', ( #23119, #19680, #25922, #40270 ), #8624, .F. ) ;
#28382=EDGE_CURVE ( 'NONE', #25632, #12844, #36035, .T. ) ;
#28401=EDGE_CURVE ( 'NONE', #42322, #29615, #18489, .T. ) ;
#28407=DIRECTION ( 'NONE',  ( 0.000000000000000000, 0.000000000000000000, 1.000000000000000000 ) ) ;
#28428=AXIS2_PLACEMENT_3D ( 'NONE', #44908, #40982, #40135 ) ;
#28465=EDGE_LOOP ( 'NONE', ( #9085, #26197, #29349, #38370 ) ) ;
#28498=DIRECTION ( 'NONE',  ( 1.000000000000000000, -0.000000000000000000, -0.000000000000000000 ) ) ;
#28501=LINE ( 'NONE', #42599, #37964 ) ;
#28519=DIRECTION ( 'NONE',  ( -0.000000000000000000, -0.000000000000000000, 1.000000000000000000 ) ) ;
#28522=ORIENTED_EDGE ( 'NONE', *, *, #23732, .F. ) ;
#28550=VECTOR ( 'NONE', #15647, 1000.000000000000000 ) ;
#28566=CARTESIAN_POINT ( 'NONE',  ( 999.9999999999992042, -590.0000000000001137, -350.0000000000000000 ) ) ;
#28580=CARTESIAN_POINT ( 'NONE',  ( 939.9999999999993179, -426.1357934546398383, 350.0000000000000000 ) ) ;
#28611=DIRECTION ( 'NONE',  ( -1.058954862565134068E-16, 0.6438296778008191223, 0.7651688349527137056 ) ) ;
#28662=CARTESIAN_POINT ( 'NONE',  ( 998.9999999999992042, 478.9999999999999432, 0.000000000000000000 ) ) ;
#28707=ORIENTED_EDGE ( 'NONE', *, *, #3269, .F. ) ;
#28717=ORIENTED_EDGE ( 'NONE', *, *, #30033, .F. ) ;
#28721=EDGE_CURVE ( 'NONE', #15902, #29488, #12901, .T. ) ;
#28752=DIRECTION ( 'NONE',  ( 1.000000000000000000, 0.000000000000000000, 0.000000000000000000 ) ) ;
#28775=CARTESIAN_POINT ( 'NONE',  ( 939.9999999999993179, -590.0000000000001137, 350.0000000000000000 ) ) ;
#28799=LINE ( 'NONE', #11244, #7723 ) ;
#28807=ORIENTED_EDGE ( 'NONE', *, *, #22728, .T. ) ;
#28866=EDGE_CURVE ( 'NONE', #23953, #20728, #26987, .T. ) ;
#28889=ORIENTED_EDGE ( 'NONE', *, *, #17866, .F. ) ;
#28896=EDGE_CURVE ( 'NONE', #28228, #37728, #25639, .T. ) ;
#28904=PLANE ( 'NONE',  #4066 ) ;
#28907=LINE ( 'NONE', #18976, #17643 ) ;
#28956=CARTESIAN_POINT ( 'NONE',  ( 914.9999999999992042, 99.99999999999984368, 360.0000000000000000 ) ) ;
#28975=CYLINDRICAL_SURFACE ( 'NONE', #7065, 7.999999999999896083 ) ;
#29014=DIRECTION ( 'NONE',  ( 0.000000000000000000, -0.6594541114781782287, 0.7517448203044211352 ) ) ;
#29062=EDGE_LOOP ( 'NONE', ( #6160, #25415, #18536, #7112 ) ) ;
#29064=CARTESIAN_POINT ( 'NONE',  ( 999.9999999999992042, -599.0000000000001137, 360.0000000000000000 ) ) ;
#29071=ORIENTED_EDGE ( 'NONE', *, *, #15946, .F. ) ;
#29073=VECTOR ( 'NONE', #32657, 1000.000000000000000 ) ;
#29087=ORIENTED_EDGE ( 'NONE', *, *, #8323, .T. ) ;
#29110=ORIENTED_EDGE ( 'NONE', *, *, #30033, .T. ) ;
#29133=CARTESIAN_POINT ( 'NONE',  ( 187.1337867209877857, 62.79977829742938411, -207.3621835540872951 ) ) ;
#29171=VECTOR ( 'NONE', #45259, 1000.000000000000000 ) ;
#29187=EDGE_CURVE ( 'NONE', #1032, #8959, #8292, .T. ) ;
#29208=FACE_OUTER_BOUND ( 'NONE', #38072, .T. ) ;
#29214=UNCERTAINTY_MEASURE_WITH_UNIT (LENGTH_MEASURE( 1.000000000000000082E-05 ), #30081, 'distance_accuracy_value', 'NONE');
#29286=ORIENTED_EDGE ( 'NONE', *, *, #29752, .F. ) ;
#29310=CARTESIAN_POINT ( 'NONE',  ( 879.9999999999992042, 249.9999999999998295, -199.9999999999999716 ) ) ;
#29329=ORIENTED_EDGE ( 'NONE', *, *, #28285, .T. ) ;
#29349=ORIENTED_EDGE ( 'NONE', *, *, #7658, .T. ) ;
#29361=EDGE_CURVE ( 'NONE', #42107, #42944, #1358, .T. ) ;
#29449=ORIENTED_EDGE ( 'NONE', *, *, #28382, .F. ) ;
#29475=EDGE_CURVE ( 'NONE', #23953, #17397, #12883, .T. ) ;
#29488=VERTEX_POINT ( 'NONE', #8964 ) ;
#29530=EDGE_CURVE ( 'NONE', #44323, #34939, #26289, .T. ) ;
#29539=DIRECTION ( 'NONE',  ( 0.000000000000000000, 1.000000000000000000, -0.000000000000000000 ) ) ;
#29565=EDGE_LOOP ( 'NONE', ( #40424, #4935, #27567, #41996 ) ) ;
#29615=VERTEX_POINT ( 'NONE', #30207 ) ;
#29624=CARTESIAN_POINT ( 'NONE',  ( 998.9999999999992042, -600.0000000000001137, -360.0000000000000000 ) ) ;
#29643=FACE_OUTER_BOUND ( 'NONE', #9659, .T. ) ;
#29649=UNCERTAINTY_MEASURE_WITH_UNIT (LENGTH_MEASURE( 1.000000000000000082E-05 ), #16477, 'distance_accuracy_value', 'NONE');
#29666=CARTESIAN_POINT ( 'NONE',  ( 927.9999999999992042, 154.9999999999998863, 350.0000000000000000 ) ) ;
#29685=DIRECTION ( 'NONE',  ( -0.000000000000000000, -0.000000000000000000, 1.000000000000000000 ) ) ;
#29738=ADVANCED_FACE ( 'NONE', ( #3413 ), #20714, .F. ) ;
#29752=EDGE_CURVE ( 'NONE', #45702, #31705, #17260, .T. ) ;
#29758=VECTOR ( 'NONE', #24580, 1000.000000000000000 ) ;
#29764=DIRECTION ( 'NONE',  ( 1.000000000000000000, 0.000000000000000000, -0.000000000000000000 ) ) ;
#29801=ADVANCED_FACE ( 'NONE', ( #31347 ), #13814, .T. ) ;
#29842=CARTESIAN_POINT ( 'NONE',  ( 914.9999999999992042, 99.99999999999984368, -350.0000000000000000 ) ) ;
#29870=PLANE ( 'NONE',  #41011 ) ;
#29887=VERTEX_POINT ( 'NONE', #20941 ) ;
#29911=VECTOR ( 'NONE', #18466, 1000.000000000000000 ) ;
#29927=LINE ( 'NONE', #2201, #38716 ) ;
#29966=VECTOR ( 'NONE', #1601, 1000.000000000000000 ) ;
#30021=AXIS2_PLACEMENT_3D ( 'NONE', #34447, #38372, #3723 ) ;
#30032=DIRECTION ( 'NONE',  ( 1.000000000000000000, 0.000000000000000000, 0.000000000000000000 ) ) ;
#30033=EDGE_CURVE ( 'NONE', #38354, #8383, #32497, .T. ) ;
#30051=PLANE ( 'NONE',  #13851 ) ;
#30052=VERTEX_POINT ( 'NONE', #28580 ) ;
#30060=EDGE_CURVE ( 'NONE', #17397, #34100, #11486, .T. ) ;
#30081=( LENGTH_UNIT ( ) NAMED_UNIT ( * ) SI_UNIT ( .MILLI., .METRE. ) );
#30098=DIRECTION ( 'NONE',  ( 0.000000000000000000, 0.000000000000000000, -1.000000000000000000 ) ) ;
#30121=PLANE ( 'NONE',  #38054 ) ;
#30132=LINE ( 'NONE', #17591, #6255 ) ;
#30135=DIRECTION ( 'NONE',  ( -0.000000000000000000, -1.000000000000000000, -0.000000000000000000 ) ) ;
#30141=CYLINDRICAL_SURFACE ( 'NONE', #4730, 1.000000000000000888 ) ;
#30172=EDGE_LOOP ( 'NONE', ( #15226, #21142, #2365, #33577, #31995, #20003 ) ) ;
#30185=LINE ( 'NONE', #33878, #35907 ) ;
#30186=LINE ( 'NONE', #19336, #28550 ) ;
#30200=APPLICATION_CONTEXT ( 'automotive_design' ) ;
#30207=CARTESIAN_POINT ( 'NONE',  ( 989.9999999999992042, -416.7569064942979935, -212.5753187112032947 ) ) ;
#30220=CARTESIAN_POINT ( 'NONE',  ( 927.9999999999992042, 154.9999999999998863, 360.0000000000000000 ) ) ;
#30229=VERTEX_POINT ( 'NONE', #21637 ) ;
#30335=ADVANCED_FACE ( 'NONE', ( #26464 ), #9134, .F. ) ;
#30341=ORIENTED_EDGE ( 'NONE', *, *, #30846, .T. ) ;
#30371=EDGE_CURVE ( 'NONE', #8196, #38417, #37542, .T. ) ;
#30420=CARTESIAN_POINT ( 'NONE',  ( 914.9999999999992042, 74.99999999999984368, -350.0000000000000000 ) ) ;
#30428=DIRECTION ( 'NONE',  ( -1.000000000000000000, -1.644774851296528363E-16, 0.000000000000000000 ) ) ;
#30441=VERTEX_POINT ( 'NONE', #5900 ) ;
#30455=CARTESIAN_POINT ( 'NONE',  ( 911.9749999999993406, 219.9999999999998863, 360.0000000000000000 ) ) ;
#30497=ORIENTED_EDGE ( 'NONE', *, *, #35423, .T. ) ;
#30510=ORIENTED_EDGE ( 'NONE', *, *, #12322, .T. ) ;
#30528=FACE_OUTER_BOUND ( 'NONE', #19493, .T. ) ;
#30545=DIRECTION ( 'NONE',  ( 0.000000000000000000, 1.000000000000000000, -0.000000000000000000 ) ) ;
#30556=VERTEX_POINT ( 'NONE', #22769 ) ;
#30569=DIRECTION ( 'NONE',  ( 0.000000000000000000, 0.000000000000000000, 1.000000000000000000 ) ) ;
#30584=CARTESIAN_POINT ( 'NONE',  ( 989.9999999999992042, -590.0000000000001137, -350.0000000000000000 ) ) ;
#30594=FACE_OUTER_BOUND ( 'NONE', #14159, .T. ) ;
#30685=CARTESIAN_POINT ( 'NONE',  ( 999.9999999999992042, -599.0000000000001137, -359.0000000000000000 ) ) ;
#30774=DIRECTION ( 'NONE',  ( 1.000000000000000000, 0.000000000000000000, 0.000000000000000000 ) ) ;
#30824=CARTESIAN_POINT ( 'NONE',  ( 998.9999999999992042, 249.9999999999998863, -359.0000000000000000 ) ) ;
#30827=ADVANCED_FACE ( 'NONE', ( #23887 ), #6121, .T. ) ;
#30830=DIRECTION ( 'NONE',  ( 1.644774851296528363E-16, -1.000000000000000000, -0.000000000000000000 ) ) ;
#30846=EDGE_CURVE ( 'NONE', #6307, #37952, #10057, .T. ) ;
#30874=DIRECTION ( 'NONE',  ( 0.000000000000000000, -1.000000000000000000, 0.000000000000000000 ) ) ;
#30877=ADVANCED_FACE ( 'NONE', ( #38454 ), #44708, .F. ) ;
#30886=CARTESIAN_POINT ( 'NONE',  ( 989.9999999999992042, -590.0000000000001137, -201.9999999999998579 ) ) ;
#30887=CONICAL_SURFACE ( 'NONE', #40518, 8.024999999999948841, 0.7853981633963380560 ) ;
#30890=CARTESIAN_POINT ( 'NONE',  ( 187.1337867209877857, 56.78581973499402835, -212.6378164459127049 ) ) ;
#30897=EDGE_CURVE ( 'NONE', #11754, #34011, #28052, .T. ) ;
#30983=CARTESIAN_POINT ( 'NONE',  ( 999.9999999999992042, 248.9999999999998863, -200.9999999999999432 ) ) ;
#31058=ADVANCED_FACE ( 'NONE', ( #29208 ), #39845, .F. ) ;
#31077=EDGE_CURVE ( 'NONE', #20728, #34100, #10711, .T. ) ;
#31092=CARTESIAN_POINT ( 'NONE',  ( 919.9999999999993179, 154.9999999999998863, 360.0000000000000000 ) ) ;
#31110=ADVANCED_FACE ( 'NONE', ( #18586 ), #4494, .F. ) ;
#31121=DIRECTION ( 'NONE',  ( 1.000000000000000000, 0.000000000000000000, -0.000000000000000000 ) ) ;
#31147=DIRECTION ( 'NONE',  ( 1.000000000000000000, 0.000000000000000000, 0.000000000000000000 ) ) ;
#31164=DIRECTION ( 'NONE',  ( 1.000000000000000000, 0.000000000000000000, -0.000000000000000000 ) ) ;
#31181=EDGE_CURVE ( 'NONE', #41469, #20456, #1015, .T. ) ;
#31185=PRODUCT_DEFINITION_CONTEXT ( 'detailed design', #18153, 'design' ) ;
#31189=CARTESIAN_POINT ( 'NONE',  ( 919.9999999999993179, 154.9999999999998863, 360.0000000000000000 ) ) ;
#31208=ORIENTED_EDGE ( 'NONE', *, *, #24136, .F. ) ;
#31243=ORIENTED_EDGE ( 'NONE', *, *, #6551, .T. ) ;
#31264=DIRECTION ( 'NONE',  ( -0.000000000000000000, -0.000000000000000000, -1.000000000000000000 ) ) ;
#31290=DIRECTION ( 'NONE',  ( 0.000000000000000000, 0.000000000000000000, -1.000000000000000000 ) ) ;
#31314=CARTESIAN_POINT ( 'NONE',  ( 939.9999999999993179, 56.78581973499407809, -212.6378164459127618 ) ) ;
#31334=CARTESIAN_POINT ( 'NONE',  ( 999.9999999999992042, 248.9999999999998863, 359.0000000000000000 ) ) ;
#31341=EDGE_LOOP ( 'NONE', ( #15310, #18381, #41477, #18335 ) ) ;
#31347=FACE_OUTER_BOUND ( 'NONE', #41199, .T. ) ;
#31356=ORIENTED_EDGE ( 'NONE', *, *, #21571, .F. ) ;
#31400=VECTOR ( 'NONE', #19787, 1000.000000000000000 ) ;
#31411=VECTOR ( 'NONE', #16017, 1000.000000000000000 ) ;
#31468=ADVANCED_FACE ( 'NONE', ( #29643 ), #29870, .T. ) ;
#31482=CIRCLE ( 'NONE', #30021, 8.024999999999948841 ) ;
#31490=ORIENTED_EDGE ( 'NONE', *, *, #29361, .T. ) ;
#31531=DIRECTION ( 'NONE',  ( 0.000000000000000000, -0.6438296778008192334, -0.7651688349527138167 ) ) ;
#31534=ORIENTED_EDGE ( 'NONE', *, *, #35423, .F. ) ;
#31535=EDGE_CURVE ( 'NONE', #36984, #38205, #13719, .T. ) ;
#31541=ORIENTED_EDGE ( 'NONE', *, *, #8626, .F. ) ;
#31573=CARTESIAN_POINT ( 'NONE',  ( 989.9999999999992042, -428.4497686941065808, 352.6378164459125060 ) ) ;
#31611=LINE ( 'NONE', #14289, #36602 ) ;
#31702=ORIENTED_EDGE ( 'NONE', *, *, #31535, .F. ) ;
#31705=VERTEX_POINT ( 'NONE', #40290 ) ;
#31723=EDGE_CURVE ( 'NONE', #25938, #15578, #12333, .T. ) ;
#31725=CARTESIAN_POINT ( 'NONE',  ( 911.9999999999994316, 154.9999999999998863, -360.0000000000000000 ) ) ;
#31734=EDGE_CURVE ( 'NONE', #41282, #5516, #8408, .T. ) ;
#31739=CARTESIAN_POINT ( 'NONE',  ( 999.9999999999992042, -590.0000000000001137, 350.0000000000000000 ) ) ;
#31743=EDGE_LOOP ( 'NONE', ( #32853, #20834, #1086, #37656 ) ) ;
#31773=CYLINDRICAL_SURFACE ( 'NONE', #7934, 1.000000000000000888 ) ;
#31775=ADVANCED_FACE ( 'NONE', ( #1463 ), #33332, .T. ) ;
#31792=PRODUCT ( 'Heavy Cast Iron Table Bed Base', 'Heavy Cast Iron Table Bed Base', '', ( #3663 ) ) ;
#31798=CARTESIAN_POINT ( 'NONE',  ( 999.9999999999992042, 249.9999999999998863, 360.0000000000000000 ) ) ;
#31828=DIRECTION ( 'NONE',  ( -1.058954862565134068E-16, 0.6438296778008191223, 0.7651688349527137056 ) ) ;
#31831=LINE ( 'NONE', #7142, #178 ) ;
#31856=ORIENTED_EDGE ( 'NONE', *, *, #960, .F. ) ;
#31883=EDGE_CURVE ( 'NONE', #16263, #30441, #44879, .T. ) ;
#31920=VERTEX_POINT ( 'NONE', #19933 ) ;
#31927=EDGE_CURVE ( 'NONE', #38417, #44323, #13007, .T. ) ;
#31975=ORIENTED_EDGE ( 'NONE', *, *, #11683, .F. ) ;
#31986=ORIENTED_EDGE ( 'NONE', *, *, #17642, .T. ) ;
#31995=ORIENTED_EDGE ( 'NONE', *, *, #37043, .T. ) ;
#32027=DIRECTION ( 'NONE',  ( 1.000000000000000000, 2.313994520913686024E-32, 2.750100768424433609E-32 ) ) ;
#32056=DIRECTION ( 'NONE',  ( -2.750100768424433062E-32, 1.672022627447525240E-16, 1.000000000000000000 ) ) ;
#32107=VECTOR ( 'NONE', #24350, 1000.000000000000000 ) ;
#32123=ORIENTED_EDGE ( 'NONE', *, *, #40670, .T. ) ;
#32146=LINE ( 'NONE', #16748, #9244 ) ;
#32172=ORIENTED_EDGE ( 'NONE', *, *, #1561, .F. ) ;
#32181=DIRECTION ( 'NONE',  ( 0.000000000000000000, 0.000000000000000000, 1.000000000000000000 ) ) ;
#32184=ORIENTED_EDGE ( 'NONE', *, *, #32833, .F. ) ;
#32186=CARTESIAN_POINT ( 'NONE',  ( 939.9999999999993179, -419.8175818341089780, -209.9999999999999716 ) ) ;
#32211=DIRECTION ( 'NONE',  ( 1.000000000000000000, 0.000000000000000000, 0.000000000000000000 ) ) ;
#32303=ORIENTED_EDGE ( 'NONE', *, *, #21571, .T. ) ;
#32305=CARTESIAN_POINT ( 'NONE',  ( 939.9999999999992042, 240.0000000000000568, -210.0000000000000000 ) ) ;
#32349=EDGE_CURVE ( 'NONE', #13695, #11328, #33234, .T. ) ;
#32362=ORIENTED_EDGE ( 'NONE', *, *, #31077, .T. ) ;
#32424=CARTESIAN_POINT ( 'NONE',  ( 939.9999999999993179, -190.2822455671962985, 69.00746428064724114 ) ) ;
#32447=CARTESIAN_POINT ( 'NONE',  ( 919.9999999999993179, 219.9999999999998863, 360.0000000000000000 ) ) ;
#32473=DIRECTION ( 'NONE',  ( 0.7071067811857625340, 0.000000000000000000, 0.7071067811873326114 ) ) ;
#32477=DIRECTION ( 'NONE',  ( 0.000000000000000000, -0.7651688349527138167, 0.6438296778008192334 ) ) ;
#32481=DIRECTION ( 'NONE',  ( -0.000000000000000000, -0.000000000000000000, 1.000000000000000000 ) ) ;
#32497=LINE ( 'NONE', #1308, #43163 ) ;
#32523=FACE_OUTER_BOUND ( 'NONE', #10390, .T. ) ;
#32551=ORIENTED_EDGE ( 'NONE', *, *, #27506, .T. ) ;
#32565=CARTESIAN_POINT ( 'NONE',  ( 989.9999999999992042, 249.9999999999998863, -209.9999999999999716 ) ) ;
#32598=DIRECTION ( 'NONE',  ( 4.625929269271485914E-16, -1.000000000000000000, 0.000000000000000000 ) ) ;
#32599=DIRECTION ( 'NONE',  ( 0.000000000000000000, -0.6594541114781790059, 0.7517448203044204691 ) ) ;
#32630=EDGE_LOOP ( 'NONE', ( #25294, #34621, #32551, #34777 ) ) ;
#32657=DIRECTION ( 'NONE',  ( -1.337618101958019798E-16, 1.000000000000000000, -1.672022627447524747E-16 ) ) ;
#32708=CARTESIAN_POINT ( 'NONE',  ( 187.1337867209877857, -428.4497686941065808, 352.6378164459125060 ) ) ;
#32711=DIRECTION ( 'NONE',  ( 1.000000000000000000, -0.000000000000000000, 0.000000000000000000 ) ) ;
#32731=CARTESIAN_POINT ( 'NONE',  ( 999.5857864376259840, 249.9999999999998863, 360.0000000000000000 ) ) ;
#32757=CARTESIAN_POINT ( 'NONE',  ( 999.9999999999992042, -599.0000000000001137, 359.0000000000000000 ) ) ;
#32760=DIRECTION ( 'NONE',  ( -1.000000000000000000, 0.000000000000000000, 0.000000000000000000 ) ) ;
#32793=CIRCLE ( 'NONE', #19483, 24.99999999999991118 ) ;
#32794=EDGE_LOOP ( 'NONE', ( #2444, #23117, #34595, #9829 ) ) ;
#32805=LINE ( 'NONE', #11104, #29966 ) ;
#32807=LINE ( 'NONE', #25864, #33437 ) ;
#32811=EDGE_CURVE ( 'NONE', #23400, #29488, #17740, .T. ) ;
#32833=EDGE_CURVE ( 'NONE', #8307, #33095, #10559, .T. ) ;
#32844=EDGE_CURVE ( 'NONE', #20464, #34629, #18184, .T. ) ;
#32853=ORIENTED_EDGE ( 'NONE', *, *, #23281, .T. ) ;
#32856=ORIENTED_EDGE ( 'NONE', *, *, #16211, .F. ) ;
#32888=ADVANCED_FACE ( 'NONE', ( #17511 ), #41765, .F. ) ;
#32893=DIRECTION ( 'NONE',  ( 0.000000000000000000, 0.000000000000000000, -1.000000000000000000 ) ) ;
#32915=ORIENTED_EDGE ( 'NONE', *, *, #1846, .T. ) ;
#32926=EDGE_CURVE ( 'NONE', #44486, #42944, #39825, .T. ) ;
#32931=DIRECTION ( 'NONE',  ( 4.625929269271485914E-16, -1.000000000000000000, -0.000000000000000000 ) ) ;
#32956=DIRECTION ( 'NONE',  ( 1.000000000000000000, 0.000000000000000000, 0.000000000000000000 ) ) ;
#33095=VERTEX_POINT ( 'NONE', #7803 ) ;
#33134=ORIENTED_EDGE ( 'NONE', *, *, #28866, .T. ) ;
#33144=ORIENTED_EDGE ( 'NONE', *, *, #12906, .T. ) ;
#33161=CARTESIAN_POINT ( 'NONE',  ( 879.9999999999990905, 50.81038600091414281, -210.0000000000000000 ) ) ;
#33179=EDGE_CURVE ( 'NONE', #42944, #26579, #43782, .T. ) ;
#33216=DIRECTION ( 'NONE',  ( 1.000000000000000000, 4.625929269271485914E-16, 0.000000000000000000 ) ) ;
#33221=CARTESIAN_POINT ( 'NONE',  ( 879.9999999999990905, 479.9999999999998863, -199.9999999999999716 ) ) ;
#33234=LINE ( 'NONE', #38627, #12263 ) ;
#33243=ORIENTED_EDGE ( 'NONE', *, *, #22728, .F. ) ;
#33300=ORIENTED_EDGE ( 'NONE', *, *, #14016, .T. ) ;
#33332=PLANE ( 'NONE',  #25517 ) ;
#33344=CARTESIAN_POINT ( 'NONE',  ( 939.9999999999992042, 74.99999999999984368, -350.0000000000000000 ) ) ;
#33356=CARTESIAN_POINT ( 'NONE',  ( 879.9999999999990905, 479.9999999999998863, -199.9999999999999716 ) ) ;
#33402=VECTOR ( 'NONE', #41448, 1000.000000000000000 ) ;
#33420=LINE ( 'NONE', #9167, #10848 ) ;
#33437=VECTOR ( 'NONE', #36490, 1000.000000000000000 ) ;
#33439=EDGE_CURVE ( 'NONE', #20663, #24719, #118, .T. ) ;
#33445=ADVANCED_FACE ( 'NONE', ( #42377, #6813, #38245 ), #10745, .F. ) ;
#33479=VERTEX_POINT ( 'NONE', #27379 ) ;
#33498=EDGE_CURVE ( 'NONE', #41469, #11754, #41938, .T. ) ;
#33501=CIRCLE ( 'NONE', #23159, 24.99999999999991118 ) ;
#33577=ORIENTED_EDGE ( 'NONE', *, *, #23732, .T. ) ;
#33614=AXIS2_PLACEMENT_3D ( 'NONE', #145, #24606, #13554 ) ;
#33636=ORIENTED_EDGE ( 'NONE', *, *, #24136, .T. ) ;
#33654=DIRECTION ( 'NONE',  ( 0.000000000000000000, 0.000000000000000000, -1.000000000000000000 ) ) ;
#33670=DIRECTION ( 'NONE',  ( 0.000000000000000000, 0.000000000000000000, 1.000000000000000000 ) ) ;
#33690=VECTOR ( 'NONE', #6892, 1000.000000000000000 ) ;
#33710=FACE_BOUND ( 'NONE', #43301, .T. ) ;
#33765=EDGE_CURVE ( 'NONE', #31920, #17901, #7739, .T. ) ;
#33809=EDGE_LOOP ( 'NONE', ( #28717, #33932, #19385, #8990 ) ) ;
#33815=CARTESIAN_POINT ( 'NONE',  ( 927.9999999999992042, 219.9999999999998863, 360.0000000000000000 ) ) ;
#33830=CARTESIAN_POINT ( 'NONE',  ( 919.9999999999993179, 219.9999999999998863, 359.9749999999999659 ) ) ;
#33849=DIRECTION ( 'NONE',  ( 0.000000000000000000, 0.7517448203044204691, 0.6594541114781790059 ) ) ;
#33866=EDGE_LOOP ( 'NONE', ( #10060, #38996, #8711, #31534 ) ) ;
#33878=CARTESIAN_POINT ( 'NONE',  ( 928.0249999999991815, 154.9999999999998863, 360.0000000000000000 ) ) ;
#33932=ORIENTED_EDGE ( 'NONE', *, *, #37641, .T. ) ;
#33997=CARTESIAN_POINT ( 'NONE',  ( 927.9999999999990905, 219.9999999999998863, -360.0000000000000000 ) ) ;
#34009=CARTESIAN_POINT ( 'NONE',  ( 989.9999999999992042, 240.0000000000001990, -201.9999999999999716 ) ) ;
#34011=VERTEX_POINT ( 'NONE', #802 ) ;
#34038=ORIENTED_EDGE ( 'NONE', *, *, #5773, .T. ) ;
#34040=MECHANICAL_DESIGN_GEOMETRIC_PRESENTATION_REPRESENTATION('',(#25201),#884);
#34047=CYLINDRICAL_SURFACE ( 'NONE', #37089, 1.000000000000000888 ) ;
#34094=DIRECTION ( 'NONE',  ( 1.258530456726092671E-16, -0.7651688349527167032, 0.6438296778008156807 ) ) ;
#34097=DIRECTION ( 'NONE',  ( 0.000000000000000000, 0.000000000000000000, 1.000000000000000000 ) ) ;
#34100=VERTEX_POINT ( 'NONE', #14447 ) ;
#34115=DIRECTION ( 'NONE',  ( 1.000000000000000000, 0.000000000000000000, 0.000000000000000000 ) ) ;
#34157=CARTESIAN_POINT ( 'NONE',  ( 939.9999999999993179, -600.0000000000001137, 350.0000000000000000 ) ) ;
#34180=LINE ( 'NONE', #6487, #11675 ) ;
#34202=DIRECTION ( 'NONE',  ( -1.000000000000000000, 0.000000000000000000, 0.000000000000000000 ) ) ;
#34218=ADVANCED_FACE ( 'NONE', ( #15569 ), #42604, .F. ) ;
#34241=DIRECTION ( 'NONE',  ( 0.000000000000000000, 0.000000000000000000, 1.000000000000000000 ) ) ;
#34267=ADVANCED_FACE ( 'NONE', ( #26850 ), #25949, .F. ) ;
#34270=DIRECTION ( 'NONE',  ( -1.000000000000000000, -4.625929269271485914E-16, 0.000000000000000000 ) ) ;
#34288=VECTOR ( 'NONE', #23134, 1000.000000000000000 ) ;
#34295=CARTESIAN_POINT ( 'NONE',  ( 879.9999999999990905, 479.9999999999998863, -210.0000000000000000 ) ) ;
#34331=DIRECTION ( 'NONE',  ( 0.000000000000000000, 0.000000000000000000, -1.000000000000000000 ) ) ;
#34388=CARTESIAN_POINT ( 'NONE',  ( 914.9999999999992042, 74.99999999999984368, 360.0000000000000000 ) ) ;
#34439=VECTOR ( 'NONE', #3147, 1000.000000000000000 ) ;
#34447=CARTESIAN_POINT ( 'NONE',  ( 919.9999999999993179, 219.9999999999998863, 360.0000000000000000 ) ) ;
#34448=AXIS2_PLACEMENT_3D ( 'NONE', #38967, #826, #35467 ) ;
#34488=ORIENTED_EDGE ( 'NONE', *, *, #36506, .T. ) ;
#34500=DIRECTION ( 'NONE',  ( 0.000000000000000000, 0.000000000000000000, 1.000000000000000000 ) ) ;
#34508=ORIENTED_EDGE ( 'NONE', *, *, #23271, .T. ) ;
#34538=EDGE_LOOP ( 'NONE', ( #19829, #3183, #5252, #40902 ) ) ;
#34550=ADVANCED_FACE ( 'NONE', ( #10004 ), #16939, .T. ) ;
#34579=VECTOR ( 'NONE', #39891, 1000.000000000000000 ) ;
#34595=ORIENTED_EDGE ( 'NONE', *, *, #15946, .T. ) ;
#34597=DIRECTION ( 'NONE',  ( 0.000000000000000000, 0.000000000000000000, 1.000000000000000000 ) ) ;
#34621=ORIENTED_EDGE ( 'NONE', *, *, #32833, .T. ) ;
#34629=VERTEX_POINT ( 'NONE', #2611 ) ;
#34672=ORIENTED_EDGE ( 'NONE', *, *, #33498, .F. ) ;
#34673=( BOUNDED_CURVE ( )  B_SPLINE_CURVE ( 3, ( #6911, #6221, #10155, #24231 ),
 .UNSPECIFIED., .F., .T. ) 
 B_SPLINE_CURVE_WITH_KNOTS ( ( 4, 4 ),
 ( 0.000000000000000000, 1.570796326794896558 ),
 .UNSPECIFIED. ) 
 CURVE ( )  GEOMETRIC_REPRESENTATION_ITEM ( )  RATIONAL_B_SPLINE_CURVE ( ( 1.000000000000000000, 0.8047378541243649375, 0.8047378541243649375, 1.000000000000000000 ) ) 
 REPRESENTATION_ITEM ( '' )  );
#34694=DIRECTION ( 'NONE',  ( 0.000000000000000000, -0.7651688349527138167, 0.6438296778008192334 ) ) ;
#34726=CARTESIAN_POINT ( 'NONE',  ( 911.9999999999993179, 219.9999999999998863, 360.0000000000000000 ) ) ;
#34777=ORIENTED_EDGE ( 'NONE', *, *, #31181, .F. ) ;
#34788=LINE ( 'NONE', #6622, #11638 ) ;
#34799=LINE ( 'NONE', #17030, #18347 ) ;
#34819=CARTESIAN_POINT ( 'NONE',  ( 998.9999999999992042, -600.0000000000001137, -360.0000000000000000 ) ) ;
#34837=CARTESIAN_POINT ( 'NONE',  ( 999.9999999999992042, 478.9999999999999432, -359.0000000000000000 ) ) ;
#34939=VERTEX_POINT ( 'NONE', #14632 ) ;
#34950=VERTEX_POINT ( 'NONE', #35387 ) ;
#34958=DIRECTION ( 'NONE',  ( -0.000000000000000000, -0.6438296778008192334, -0.7651688349527135946 ) ) ;
#34989=DIRECTION ( 'NONE',  ( 1.000000000000000000, 0.000000000000000000, -0.000000000000000000 ) ) ;
#35013=LINE ( 'NONE', #42402, #19675 ) ;
#35084=AXIS2_PLACEMENT_3D ( 'NONE', #10026, #41438, #24092 ) ;
#35159=VECTOR ( 'NONE', #82, 1000.000000000000000 ) ;
#35256=DIRECTION ( 'NONE',  ( 1.000000000000000000, 0.000000000000000000, 0.000000000000000000 ) ) ;
#35387=CARTESIAN_POINT ( 'NONE',  ( 989.9999999999992042, 46.15097736693707020, 350.0000000000000000 ) ) ;
#35401=ADVANCED_FACE ( 'NONE', ( #15969 ), #30051, .T. ) ;
#35418=DIRECTION ( 'NONE',  ( -0.000000000000000000, 1.000000000000000000, -0.000000000000000000 ) ) ;
#35423=EDGE_CURVE ( 'NONE', #30052, #14449, #19655, .T. ) ;
#35428=DIRECTION ( 'NONE',  ( 0.000000000000000000, 0.000000000000000000, 1.000000000000000000 ) ) ;
#35459=CARTESIAN_POINT ( 'NONE',  ( 939.9999999999993179, -414.5899773927343404, -210.0000000000000000 ) ) ;
#35467=DIRECTION ( 'NONE',  ( 0.000000000000000000, 0.000000000000000000, -1.000000000000000000 ) ) ;
#35468=CARTESIAN_POINT ( 'NONE',  ( 939.9999999999992042, 74.99999999999984368, 350.0000000000000000 ) ) ;
#35522=DIRECTION ( 'NONE',  ( -1.000000000000000000, 0.000000000000000000, 0.000000000000000000 ) ) ;
#35566=CYLINDRICAL_SURFACE ( 'NONE', #44712, 1.000000000000000888 ) ;
#35573=AXIS2_PLACEMENT_3D ( 'NONE', #13108, #34097, #9633 ) ;
#35612=ORIENTED_EDGE ( 'NONE', *, *, #19626, .F. ) ;
#35637=LINE ( 'NONE', #39823, #18731 ) ;
#35641=EDGE_CURVE ( 'NONE', #13352, #28228, #34180, .T. ) ;
#35659=DIRECTION ( 'NONE',  ( -1.000000000000000000, 0.000000000000000000, 0.000000000000000000 ) ) ;
#35670=ORIENTED_EDGE ( 'NONE', *, *, #1561, .T. ) ;
#35692=CARTESIAN_POINT ( 'NONE',  ( 928.0249999999991815, 219.9999999999998863, 360.0000000000000000 ) ) ;
#35701=DIRECTION ( 'NONE',  ( 1.000000000000000000, 0.000000000000000000, 0.000000000000000000 ) ) ;
#35704=EDGE_CURVE ( 'NONE', #41166, #30229, #14655, .T. ) ;
#35729=CARTESIAN_POINT ( 'NONE',  ( 999.9999999999992042, 248.9999999999998863, 359.0000000000000000 ) ) ;
#35758=CARTESIAN_POINT ( 'NONE',  ( 187.1337867209877857, 62.79977829742938411, -207.3621835540872951 ) ) ;
#35787=AXIS2_PLACEMENT_3D ( 'NONE', #42911, #32056, #195 ) ;
#35810=ORIENTED_EDGE ( 'NONE', *, *, #38468, .T. ) ;
#35834=VECTOR ( 'NONE', #38181, 1000.000000000000000 ) ;
#35840=VECTOR ( 'NONE', #9622, 1000.000000000000000 ) ;
#35907=VECTOR ( 'NONE', #2230, 999.9999999999998863 ) ;
#35912=EDGE_CURVE ( 'NONE', #966, #13695, #41943, .T. ) ;
#35913=ORIENTED_EDGE ( 'NONE', *, *, #3573, .T. ) ;
#35995=LINE ( 'NONE', #29064, #8617 ) ;
#35996=LINE ( 'NONE', #4361, #39614 ) ;
#36032=EDGE_CURVE ( 'NONE', #22430, #25938, #34799, .T. ) ;
#36035=LINE ( 'NONE', #32565, #42357 ) ;
#36046=EDGE_LOOP ( 'NONE', ( #27545, #10707, #2157, #15008 ) ) ;
#36117=CARTESIAN_POINT ( 'NONE',  ( 939.9999999999992042, 240.0000000000000568, -201.9999999999999716 ) ) ;
#36124=ORIENTED_EDGE ( 'NONE', *, *, #41125, .F. ) ;
#36153=CARTESIAN_POINT ( 'NONE',  ( 939.9999999999992042, 240.0000000000000568, -201.9999999999999716 ) ) ;
#36158=LINE ( 'NONE', #35692, #14482 ) ;
#36165=DIRECTION ( 'NONE',  ( -0.000000000000000000, -1.000000000000000000, -0.000000000000000000 ) ) ;
#36212=CARTESIAN_POINT ( 'NONE',  ( 999.5857864376259840, -600.0000000000001137, 360.0000000000000000 ) ) ;
#36213=LINE ( 'NONE', #22335, #37374 ) ;
#36265=VECTOR ( 'NONE', #9641, 1000.000000000000000 ) ;
#36284=DIRECTION ( 'NONE',  ( 1.000000000000000000, 4.625929269271485914E-16, 0.000000000000000000 ) ) ;
#36291=CIRCLE ( 'NONE', #41473, 8.000000000000007105 ) ;
#36344=ORIENTED_EDGE ( 'NONE', *, *, #10062, .F. ) ;
#36377=CARTESIAN_POINT ( 'NONE',  ( 919.9999999999993179, 154.9999999999998863, -350.0000000000000000 ) ) ;
#36473=DIRECTION ( 'NONE',  ( -1.644774851296528363E-16, 1.000000000000000000, 0.000000000000000000 ) ) ;
#36484=ORIENTED_EDGE ( 'NONE', *, *, #44388, .T. ) ;
#36490=DIRECTION ( 'NONE',  ( 1.644774851296528363E-16, -1.000000000000000000, -0.000000000000000000 ) ) ;
#36506=EDGE_CURVE ( 'NONE', #15902, #16465, #39672, .T. ) ;
#36510=FACE_OUTER_BOUND ( 'NONE', #33866, .T. ) ;
#36568=CARTESIAN_POINT ( 'NONE',  ( 989.9999999999992042, 249.9999999999998863, 350.0000000000000000 ) ) ;
#36602=VECTOR ( 'NONE', #41789, 1000.000000000000000 ) ;
#36640=CARTESIAN_POINT ( 'NONE',  ( 939.9999999999992042, 56.73212367640090292, 362.5753187112032947 ) ) ;
#36687=ORIENTED_EDGE ( 'NONE', *, *, #11683, .T. ) ;
#36708=ORIENTED_EDGE ( 'NONE', *, *, #29361, .F. ) ;
#36740=EDGE_CURVE ( 'NONE', #5516, #12844, #11708, .T. ) ;
#36751=AXIS2_PLACEMENT_3D ( 'NONE', #42951, #28407, #21703 ) ;
#36761=ORIENTED_EDGE ( 'NONE', *, *, #15671, .T. ) ;
#36784=CIRCLE ( 'NONE', #658, 7.999999999999785061 ) ;
#36790=PLANE ( 'NONE',  #18058 ) ;
#36844=DIRECTION ( 'NONE',  ( 0.000000000000000000, -0.7517448203044211352, -0.6594541114781782287 ) ) ;
#36847=EDGE_CURVE ( 'NONE', #9644, #6307, #36784, .T. ) ;
#36904=FACE_BOUND ( 'NONE', #44910, .T. ) ;
#36945=ORIENTED_EDGE ( 'NONE', *, *, #13086, .F. ) ;
#36966=PLANE ( 'NONE',  #35787 ) ;
#36979=ORIENTED_EDGE ( 'NONE', *, *, #20723, .T. ) ;
#36984=VERTEX_POINT ( 'NONE', #33997 ) ;
#37003=CARTESIAN_POINT ( 'NONE',  ( 919.9999999999993179, 219.9999999999998863, 359.9749999999999659 ) ) ;
#37027=ORIENTED_EDGE ( 'NONE', *, *, #40217, .F. ) ;
#37034=ORIENTED_EDGE ( 'NONE', *, *, #11041, .F. ) ;
#37043=EDGE_CURVE ( 'NONE', #8196, #14052, #2826, .T. ) ;
#37058=VECTOR ( 'NONE', #33216, 1000.000000000000000 ) ;
#37089=AXIS2_PLACEMENT_3D ( 'NONE', #30824, #26658, #26445 ) ;
#37098=DIRECTION ( 'NONE',  ( 1.000000000000000000, 0.000000000000000000, -0.000000000000000000 ) ) ;
#37238=VECTOR ( 'NONE', #32893, 1000.000000000000000 ) ;
#37257=DIRECTION ( 'NONE',  ( 0.000000000000000000, 0.000000000000000000, 1.000000000000000000 ) ) ;
#37294=VECTOR ( 'NONE', #43259, 1000.000000000000000 ) ;
#37296=DIRECTION ( 'NONE',  ( -1.000000000000000000, 0.000000000000000000, 0.000000000000000000 ) ) ;
#37332=ORIENTED_EDGE ( 'NONE', *, *, #19126, .F. ) ;
#37374=VECTOR ( 'NONE', #28611, 1000.000000000000114 ) ;
#37460=DIRECTION ( 'NONE',  ( -1.000000000000000000, -1.644774851296528363E-16, 0.000000000000000000 ) ) ;
#37465=ADVANCED_FACE ( 'NONE', ( #8132 ), #30887, .F. ) ;
#37502=ORIENTED_EDGE ( 'NONE', *, *, #35704, .F. ) ;
#37509=CARTESIAN_POINT ( 'NONE',  ( 914.9999999999992042, 74.99999999999984368, -360.0000000000000000 ) ) ;
#37515=ORIENTED_EDGE ( 'NONE', *, *, #29530, .T. ) ;
#37522=LINE ( 'NONE', #5406, #16370 ) ;
#37542=LINE ( 'NONE', #1973, #45407 ) ;
#37639=CARTESIAN_POINT ( 'NONE',  ( 914.9999999999992042, 99.99999999999984368, 350.0000000000000000 ) ) ;
#37641=EDGE_CURVE ( 'NONE', #38354, #15902, #28907, .T. ) ;
#37656=ORIENTED_EDGE ( 'NONE', *, *, #352, .F. ) ;
#37728=VERTEX_POINT ( 'NONE', #8799 ) ;
#37778=VECTOR ( 'NONE', #34270, 1000.000000000000000 ) ;
#37805=LINE ( 'NONE', #6154, #9356 ) ;
#37820=ORIENTED_EDGE ( 'NONE', *, *, #2582, .T. ) ;
#37829=AXIS2_PLACEMENT_3D ( 'NONE', #32708, #29014, #36844 ) ;
#37861=CIRCLE ( 'NONE', #23821, 7.999999999999896083 ) ;
#37872=CARTESIAN_POINT ( 'NONE',  ( 939.9999999999993179, -418.3138125091625170, -201.9999999999998863 ) ) ;
#37923=VECTOR ( 'NONE', #25032, 1000.000000000000000 ) ;
#37952=VERTEX_POINT ( 'NONE', #40658 ) ;
#37964=VECTOR ( 'NONE', #10960, 1000.000000000000000 ) ;
#37975=VERTEX_POINT ( 'NONE', #40445 ) ;
#37978=VECTOR ( 'NONE', #43117, 1000.000000000000000 ) ;
#38019=ORIENTED_EDGE ( 'NONE', *, *, #16727, .T. ) ;
#38054=AXIS2_PLACEMENT_3D ( 'NONE', #12568, #25965, #1935 ) ;
#38072=EDGE_LOOP ( 'NONE', ( #15685, #26802, #1488, #31208 ) ) ;
#38123=CONICAL_SURFACE ( 'NONE', #21898, 8.024999999999948841, 0.7853981633963380560 ) ;
#38137=ORIENTED_EDGE ( 'NONE', *, *, #2079, .F. ) ;
#38181=DIRECTION ( 'NONE',  ( 0.000000000000000000, -1.000000000000000000, 1.672022627447524993E-16 ) ) ;
#38205=VERTEX_POINT ( 'NONE', #39037 ) ;
#38245=FACE_OUTER_BOUND ( 'NONE', #7992, .T. ) ;
#38247=VERTEX_POINT ( 'NONE', #41813 ) ;
#38294=DIRECTION ( 'NONE',  ( 0.000000000000000000, -0.000000000000000000, 1.000000000000000000 ) ) ;
#38324=CARTESIAN_POINT ( 'NONE',  ( 914.9999999999992042, 74.99999999999984368, 360.0000000000000000 ) ) ;
#38354=VERTEX_POINT ( 'NONE', #27709 ) ;
#38370=ORIENTED_EDGE ( 'NONE', *, *, #44398, .T. ) ;
#38372=DIRECTION ( 'NONE',  ( -0.000000000000000000, -0.000000000000000000, 1.000000000000000000 ) ) ;
#38417=VERTEX_POINT ( 'NONE', #17557 ) ;
#38454=FACE_OUTER_BOUND ( 'NONE', #32630, .T. ) ;
#38468=EDGE_CURVE ( 'NONE', #13695, #966, #44195, .T. ) ;
#38480=EDGE_LOOP ( 'NONE', ( #7873, #80, #18920, #43365 ) ) ;
#38508=CARTESIAN_POINT ( 'NONE',  ( 506.1531787467675940, 50.81038600091411439, -217.3872392842761769 ) ) ;
#38511=ADVANCED_FACE ( 'NONE', ( #32523 ), #9338, .F. ) ;
#38543=DIRECTION ( 'NONE',  ( -0.000000000000000000, -0.000000000000000000, -1.000000000000000000 ) ) ;
#38617=PLANE ( 'NONE',  #40954 ) ;
#38627=CARTESIAN_POINT ( 'NONE',  ( 927.9999999999992042, 219.9999999999998863, 360.0000000000000000 ) ) ;
#38647=ORIENTED_EDGE ( 'NONE', *, *, #24398, .T. ) ;
#38671=LINE ( 'NONE', #10039, #2657 ) ;
#38674=DIRECTION ( 'NONE',  ( 0.000000000000000000, -0.7651688349527138167, 0.6438296778008192334 ) ) ;
#38683=VECTOR ( 'NONE', #2888, 1000.000000000000000 ) ;
#38685=EDGE_CURVE ( 'NONE', #33479, #2741, #1332, .T. ) ;
#38689=DIRECTION ( 'NONE',  ( 0.000000000000000000, -0.7651688349527138167, 0.6438296778008192334 ) ) ;
#38707=ORIENTED_EDGE ( 'NONE', *, *, #33498, .T. ) ;
#38709=VECTOR ( 'NONE', #30428, 1000.000000000000000 ) ;
#38716=VECTOR ( 'NONE', #26461, 1000.000000000000000 ) ;
#38717=ORIENTED_EDGE ( 'NONE', *, *, #11041, .T. ) ;
#38723=CYLINDRICAL_SURFACE ( 'NONE', #21049, 7.999999999999896083 ) ;
#38754=ORIENTED_EDGE ( 'NONE', *, *, #13551, .F. ) ;
#38757=CARTESIAN_POINT ( 'NONE',  ( 919.9999999999993179, 219.9999999999998863, -350.0000000000000000 ) ) ;
#38766=AXIS2_PLACEMENT_3D ( 'NONE', #12626, #26704, #23232 ) ;
#38906=DIRECTION ( 'NONE',  ( 0.000000000000000000, 0.000000000000000000, -1.000000000000000000 ) ) ;
#38967=CARTESIAN_POINT ( 'NONE',  ( 879.9999999999992042, 99.99999999999984368, 360.0000000000000000 ) ) ;
#38996=ORIENTED_EDGE ( 'NONE', *, *, #15433, .F. ) ;
#39037=CARTESIAN_POINT ( 'NONE',  ( 911.9999999999994316, 219.9999999999998863, -360.0000000000000000 ) ) ;
#39111=ORIENTED_EDGE ( 'NONE', *, *, #44388, .F. ) ;
#39137=LINE ( 'NONE', #7487, #28113 ) ;
#39289=EDGE_LOOP ( 'NONE', ( #37515, #22627, #43132, #25163 ) ) ;
#39413=CARTESIAN_POINT ( 'NONE',  ( 919.9999999999993179, 154.9999999999998863, 360.0000000000000000 ) ) ;
#39431=EDGE_CURVE ( 'NONE', #34950, #15624, #18340, .T. ) ;
#39435=( GEOMETRIC_REPRESENTATION_CONTEXT ( 3 ) GLOBAL_UNCERTAINTY_ASSIGNED_CONTEXT ( ( #29649 ) ) GLOBAL_UNIT_ASSIGNED_CONTEXT ( ( #16477, #40520, #9086 ) ) REPRESENTATION_CONTEXT ( 'NONE', 'WORKASPACE' ) );
#39442=ORIENTED_EDGE ( 'NONE', *, *, #30060, .F. ) ;
#39450=VECTOR ( 'NONE', #25394, 1000.000000000000000 ) ;
#39472=AXIS2_PLACEMENT_3D ( 'NONE', #4016, #39601, #7957 ) ;
#39489=AXIS2_PLACEMENT_3D ( 'NONE', #17443, #35428, #18126 ) ;
#39552=DIRECTION ( 'NONE',  ( 1.000000000000000000, 0.000000000000000000, 0.000000000000000000 ) ) ;
#39601=DIRECTION ( 'NONE',  ( 0.000000000000000000, 0.000000000000000000, 1.000000000000000000 ) ) ;
#39614=VECTOR ( 'NONE', #33654, 1000.000000000000000 ) ;
#39622=VERTEX_POINT ( 'NONE', #29842 ) ;
#39629=EDGE_LOOP ( 'NONE', ( #17045, #26417, #26298, #18490, #25751, #38754, #21487, #39768, #25178, #6415, #43516, #10243 ) ) ;
#39643=LINE ( 'NONE', #36153, #3404 ) ;
#39672=LINE ( 'NONE', #25091, #26426 ) ;
#39707=DIRECTION ( 'NONE',  ( 0.000000000000000000, -0.6594541114781790059, 0.7517448203044204691 ) ) ;
#39748=CARTESIAN_POINT ( 'NONE',  ( 187.1337867209877857, -416.7569064942979935, -212.5753187112033231 ) ) ;
#39749=ORIENTED_EDGE ( 'NONE', *, *, #36740, .T. ) ;
#39768=ORIENTED_EDGE ( 'NONE', *, *, #19956, .T. ) ;
#39801=ORIENTED_EDGE ( 'NONE', *, *, #6921, .T. ) ;
#39823=CARTESIAN_POINT ( 'NONE',  ( 914.9999999999992042, -431.4567479753239354, 350.0000000000000000 ) ) ;
#39825=( BOUNDED_CURVE ( )  B_SPLINE_CURVE ( 3, ( #35729, #8033, #32731, #7567 ),
 .UNSPECIFIED., .F., .T. ) 
 B_SPLINE_CURVE_WITH_KNOTS ( ( 4, 4 ),
 ( 1.570796326794896558, 3.141592653589793116 ),
 .UNSPECIFIED. ) 
 CURVE ( )  GEOMETRIC_REPRESENTATION_ITEM ( )  RATIONAL_B_SPLINE_CURVE ( ( 1.000000000000000000, 0.8047378541243649375, 0.8047378541243649375, 1.000000000000000000 ) ) 
 REPRESENTATION_ITEM ( '' )  );
#39839=LINE ( 'NONE', #18803, #37238 ) ;
#39844=DIRECTION ( 'NONE',  ( -0.000000000000000000, -0.000000000000000000, 1.000000000000000000 ) ) ;
#39845=CYLINDRICAL_SURFACE ( 'NONE', #20292, 7.999999999999896083 ) ;
#39851=EDGE_CURVE ( 'NONE', #41554, #10806, #267, .T. ) ;
#39890=CARTESIAN_POINT ( 'NONE',  ( 911.9999999999993179, 219.9999999999998863, -350.0000000000000000 ) ) ;
#39891=DIRECTION ( 'NONE',  ( 1.000000000000000000, 4.625929269271485914E-16, 0.000000000000000000 ) ) ;
#39929=DIRECTION ( 'NONE',  ( 0.000000000000000000, -0.000000000000000000, 1.000000000000000000 ) ) ;
#39964=EDGE_CURVE ( 'NONE', #4785, #9965, #10411, .T. ) ;
#39974=LINE ( 'NONE', #11571, #6173 ) ;
#40038=LINE ( 'NONE', #36117, #29073 ) ;
#40076=AXIS2_PLACEMENT_3D ( 'NONE', #33221, #27192, #16576 ) ;
#40135=DIRECTION ( 'NONE',  ( 1.000000000000000000, 0.000000000000000000, 0.000000000000000000 ) ) ;
#40177=ORIENTED_EDGE ( 'NONE', *, *, #43330, .T. ) ;
#40179=CIRCLE ( 'NONE', #20253, 8.000000000000007105 ) ;
#40187=ORIENTED_EDGE ( 'NONE', *, *, #31535, .T. ) ;
#40217=EDGE_CURVE ( 'NONE', #14175, #24400, #31482, .T. ) ;
#40251=EDGE_LOOP ( 'NONE', ( #16482, #13707, #407, #12237 ) ) ;
#40261=AXIS2_PLACEMENT_3D ( 'NONE', #39413, #11691, #25764 ) ;
#40270=FACE_OUTER_BOUND ( 'NONE', #5640, .T. ) ;
#40275=DIRECTION ( 'NONE',  ( -4.625929269271485914E-16, 1.000000000000000000, 0.000000000000000000 ) ) ;
#40290=CARTESIAN_POINT ( 'NONE',  ( 939.9999999999993179, -590.0000000000001137, -350.0000000000000000 ) ) ;
#40301=ORIENTED_EDGE ( 'NONE', *, *, #22159, .F. ) ;
#40303=VECTOR ( 'NONE', #28115, 1000.000000000000000 ) ;
#40305=ORIENTED_EDGE ( 'NONE', *, *, #17027, .F. ) ;
#40320=VERTEX_POINT ( 'NONE', #7641 ) ;
#40368=VECTOR ( 'NONE', #11163, 1000.000000000000114 ) ;
#40382=CARTESIAN_POINT ( 'NONE',  ( 998.9999999999992042, -600.0000000000001137, 360.0000000000000000 ) ) ;
#40424=ORIENTED_EDGE ( 'NONE', *, *, #39851, .T. ) ;
#40445=CARTESIAN_POINT ( 'NONE',  ( 989.9999999999992042, -590.0000000000001137, 350.0000000000000000 ) ) ;
#40486=VECTOR ( 'NONE', #1513, 1000.000000000000114 ) ;
#40507=DIRECTION ( 'NONE',  ( 0.000000000000000000, 0.7651688349527167032, -0.6438296778008156807 ) ) ;
#40518=AXIS2_PLACEMENT_3D ( 'NONE', #4646, #4874, #18522 ) ;
#40520=( NAMED_UNIT ( * ) PLANE_ANGLE_UNIT ( ) SI_UNIT ( $, .RADIAN. ) );
#40532=DIRECTION ( 'NONE',  ( -0.000000000000000000, -0.000000000000000000, -1.000000000000000000 ) ) ;
#40538=CARTESIAN_POINT ( 'NONE',  ( 914.9999999999992042, 99.99999999999984368, 360.0000000000000000 ) ) ;
#40549=DIRECTION ( 'NONE',  ( -0.000000000000000000, -0.6438296778008192334, -0.7651688349527135946 ) ) ;
#40595=CARTESIAN_POINT ( 'NONE',  ( 939.9999999999993179, 50.81038600091411439, -193.6948738798775764 ) ) ;
#40658=CARTESIAN_POINT ( 'NONE',  ( 911.9999999999993179, 154.9999999999998863, -350.0000000000000000 ) ) ;
#40670=EDGE_CURVE ( 'NONE', #24400, #14175, #27533, .T. ) ;
#40745=ORIENTED_EDGE ( 'NONE', *, *, #19126, .T. ) ;
#40756=EDGE_CURVE ( 'NONE', #34100, #30229, #39974, .T. ) ;
#40796=ORIENTED_EDGE ( 'NONE', *, *, #17027, .T. ) ;
#40816=EDGE_CURVE ( 'NONE', #6488, #1032, #32807, .T. ) ;
#40848=VERTEX_POINT ( 'NONE', #12016 ) ;
#40866=PLANE ( 'NONE',  #1274 ) ;
#40902=ORIENTED_EDGE ( 'NONE', *, *, #35641, .F. ) ;
#40950=CARTESIAN_POINT ( 'NONE',  ( 879.9999999999992042, 239.9999999999998010, 360.0000000000000000 ) ) ;
#40954=AXIS2_PLACEMENT_3D ( 'NONE', #27764, #34694, #10210 ) ;
#40982=DIRECTION ( 'NONE',  ( -0.000000000000000000, -0.000000000000000000, 1.000000000000000000 ) ) ;
#40983=LINE ( 'NONE', #27125, #7119 ) ;
#40987=FACE_OUTER_BOUND ( 'NONE', #4961, .T. ) ;
#40992=FACE_OUTER_BOUND ( 'NONE', #34538, .T. ) ;
#40997=VECTOR ( 'NONE', #21330, 1000.000000000000000 ) ;
#41011=AXIS2_PLACEMENT_3D ( 'NONE', #15350, #30098, #43503 ) ;
#41015=VERTEX_POINT ( 'NONE', #17292 ) ;
#41059=FACE_OUTER_BOUND ( 'NONE', #31743, .T. ) ;
#41087=DIRECTION ( 'NONE',  ( -0.000000000000000000, -0.000000000000000000, 1.000000000000000000 ) ) ;
#41125=EDGE_CURVE ( 'NONE', #5691, #6488, #17223, .T. ) ;
#41166=VERTEX_POINT ( 'NONE', #6671 ) ;
#41199=EDGE_LOOP ( 'NONE', ( #43784, #33243, #36344, #13483 ) ) ;
#41236=CARTESIAN_POINT ( 'NONE',  ( 939.9999999999993179, -590.0000000000001137, 360.0000000000000000 ) ) ;
#41238=ADVANCED_FACE ( 'NONE', ( #27453 ), #23976, .F. ) ;
#41282=VERTEX_POINT ( 'NONE', #44327 ) ;
#41285=FACE_OUTER_BOUND ( 'NONE', #920, .T. ) ;
#41290=CARTESIAN_POINT ( 'NONE',  ( 911.9749999999993406, 219.9999999999998863, 360.0000000000000000 ) ) ;
#41313=ORIENTED_EDGE ( 'NONE', *, *, #25587, .T. ) ;
#41328=LINE ( 'NONE', #2279, #45498 ) ;
#41385=LINE ( 'NONE', #9732, #45501 ) ;
#41399=CARTESIAN_POINT ( 'NONE',  ( 919.9999999999993179, 219.9999999999998863, 360.0000000000000000 ) ) ;
#41423=EDGE_LOOP ( 'NONE', ( #6542, #44521, #26307, #23276 ) ) ;
#41424=SHAPE_REPRESENTATION_RELATIONSHIP ( 'NONE' , 'NONE' ,  #10941, #27670 ) ;
#41438=DIRECTION ( 'NONE',  ( 0.000000000000000000, 1.000000000000000000, -0.000000000000000000 ) ) ;
#41443=DIRECTION ( 'NONE',  ( 0.000000000000000000, 0.000000000000000000, -1.000000000000000000 ) ) ;
#41447=LINE ( 'NONE', #25924, #21584 ) ;
#41448=DIRECTION ( 'NONE',  ( 1.644774851296528363E-16, -1.000000000000000000, 0.000000000000000000 ) ) ;
#41454=CARTESIAN_POINT ( 'NONE',  ( 911.9999999999993179, 219.9999999999998863, 350.0000000000000000 ) ) ;
#41469=VERTEX_POINT ( 'NONE', #21446 ) ;
#41473=AXIS2_PLACEMENT_3D ( 'NONE', #33830, #44222, #16052 ) ;
#41477=ORIENTED_EDGE ( 'NONE', *, *, #693, .F. ) ;
#41554=VERTEX_POINT ( 'NONE', #10362 ) ;
#41564=EDGE_CURVE ( 'NONE', #861, #29887, #31831, .T. ) ;
#41594=ADVANCED_FACE ( 'NONE', ( #4364 ), #24438, .F. ) ;
#41639=ORIENTED_EDGE ( 'NONE', *, *, #4887, .T. ) ;
#41717=EDGE_CURVE ( 'NONE', #30556, #10806, #25606, .T. ) ;
#41735=CARTESIAN_POINT ( 'NONE',  ( 879.9999999999992042, 249.9999999999998295, 360.0000000000000000 ) ) ;
#41755=ORIENTED_EDGE ( 'NONE', *, *, #16194, .F. ) ;
#41765=CYLINDRICAL_SURFACE ( 'NONE', #9849, 7.999999999999896083 ) ;
#41789=DIRECTION ( 'NONE',  ( -1.000000000000000000, 0.000000000000000000, 0.000000000000000000 ) ) ;
#41792=CARTESIAN_POINT ( 'NONE',  ( 919.9999999999993179, 154.9999999999998863, 360.0000000000000000 ) ) ;
#41813=CARTESIAN_POINT ( 'NONE',  ( 989.9999999999992042, 239.9999999999998863, 350.0000000000000000 ) ) ;
#41829=DIRECTION ( 'NONE',  ( 1.000000000000000000, 0.000000000000000000, 0.000000000000000000 ) ) ;
#41833=AXIS2_PLACEMENT_3D ( 'NONE', #25817, #32760, #8505 ) ;
#41841=ORIENTED_EDGE ( 'NONE', *, *, #32811, .F. ) ;
#41847=ORIENTED_EDGE ( 'NONE', *, *, #11703, .T. ) ;
#41905=DIRECTION ( 'NONE',  ( -1.000000000000000000, 0.000000000000000000, -0.000000000000000000 ) ) ;
#41938=LINE ( 'NONE', #10504, #29758 ) ;
#41943=CIRCLE ( 'NONE', #36751, 7.999999999999896083 ) ;
#41996=ORIENTED_EDGE ( 'NONE', *, *, #23271, .F. ) ;
#42071=CARTESIAN_POINT ( 'NONE',  ( 911.9999999999993179, 154.9999999999998863, 350.0000000000000000 ) ) ;
#42107=VERTEX_POINT ( 'NONE', #9170 ) ;
#42141=EDGE_CURVE ( 'NONE', #34629, #20464, #6834, .T. ) ;
#42145=DIRECTION ( 'NONE',  ( 1.000000000000000000, -0.000000000000000000, 0.000000000000000000 ) ) ;
#42146=DIRECTION ( 'NONE',  ( -0.000000000000000000, 0.000000000000000000, -1.000000000000000000 ) ) ;
#42180=FACE_OUTER_BOUND ( 'NONE', #27549, .T. ) ;
#42199=VECTOR ( 'NONE', #17019, 1000.000000000000000 ) ;
#42291=AXIS2_PLACEMENT_3D ( 'NONE', #6128, #3364, #34989 ) ;
#42298=DIRECTION ( 'NONE',  ( -0.000000000000000000, -0.000000000000000000, 1.000000000000000000 ) ) ;
#42322=VERTEX_POINT ( 'NONE', #6404 ) ;
#42328=ORIENTED_EDGE ( 'NONE', *, *, #6905, .F. ) ;
#42336=ORIENTED_EDGE ( 'NONE', *, *, #44180, .F. ) ;
#42340=AXIS2_PLACEMENT_3D ( 'NONE', #5415, #29685, #5201 ) ;
#42357=VECTOR ( 'NONE', #11317, 1000.000000000000000 ) ;
#42377=FACE_BOUND ( 'NONE', #5085, .T. ) ;
#42402=CARTESIAN_POINT ( 'NONE',  ( 187.1337867209877857, -190.2822455671962985, 69.00746428064726956 ) ) ;
#42489=VECTOR ( 'NONE', #16445, 1000.000000000000000 ) ;
#42525=ORIENTED_EDGE ( 'NONE', *, *, #39431, .T. ) ;
#42534=DIRECTION ( 'NONE',  ( 0.000000000000000000, 0.000000000000000000, -1.000000000000000000 ) ) ;
#42550=PRODUCT_DEFINITION ( 'UNKNOWN', '', #9073, #31185 ) ;
#42593=DIRECTION ( 'NONE',  ( 1.000000000000000000, -0.000000000000000000, -0.000000000000000000 ) ) ;
#42599=CARTESIAN_POINT ( 'NONE',  ( 989.9999999999992042, 240.0000000000001990, -201.9999999999999716 ) ) ;
#42604=CONICAL_SURFACE ( 'NONE', #44064, 8.024999999999948841, 0.7853981633963380560 ) ;
#42647=DIRECTION ( 'NONE',  ( -0.000000000000000000, -0.000000000000000000, -1.000000000000000000 ) ) ;
#42911=CARTESIAN_POINT ( 'NONE',  ( 1820.038553321469863, 240.0000000000001990, -201.9999999999999716 ) ) ;
#42914=DIRECTION ( 'NONE',  ( 0.000000000000000000, 0.000000000000000000, -1.000000000000000000 ) ) ;
#42944=VERTEX_POINT ( 'NONE', #25978 ) ;
#42949=VECTOR ( 'NONE', #831, 1000.000000000000000 ) ;
#42951=CARTESIAN_POINT ( 'NONE',  ( 919.9999999999993179, 219.9999999999998863, 350.0000000000000000 ) ) ;
#42991=ADVANCED_FACE ( 'NONE', ( #15160 ), #18621, .T. ) ;
#43014=ORIENTED_EDGE ( 'NONE', *, *, #32844, .F. ) ;
#43061=ADVANCED_FACE ( 'NONE', ( #40992 ), #34047, .T. ) ;
#43117=DIRECTION ( 'NONE',  ( -0.000000000000000000, -0.000000000000000000, 1.000000000000000000 ) ) ;
#43126=VECTOR ( 'NONE', #29764, 1000.000000000000000 ) ;
#43132=ORIENTED_EDGE ( 'NONE', *, *, #22159, .T. ) ;
#43163=VECTOR ( 'NONE', #32027, 1000.000000000000000 ) ;
#43259=DIRECTION ( 'NONE',  ( 1.000000000000000000, 4.625929269271485914E-16, 0.000000000000000000 ) ) ;
#43287=DIRECTION ( 'NONE',  ( 1.000000000000000000, 0.000000000000000000, -0.000000000000000000 ) ) ;
#43301=EDGE_LOOP ( 'NONE', ( #11880, #8240 ) ) ;
#43325=CARTESIAN_POINT ( 'NONE',  ( 879.9999999999992042, 99.99999999999984368, 360.0000000000000000 ) ) ;
#43330=EDGE_CURVE ( 'NONE', #44486, #11392, #20191, .T. ) ;
#43343=EDGE_CURVE ( 'NONE', #27904, #30052, #5882, .T. ) ;
#43365=ORIENTED_EDGE ( 'NONE', *, *, #16194, .T. ) ;
#43382=LINE ( 'NONE', #11750, #25615 ) ;
#43414=EDGE_LOOP ( 'NONE', ( #65, #1989 ) ) ;
#43437=DIRECTION ( 'NONE',  ( 0.000000000000000000, 1.000000000000000000, -0.000000000000000000 ) ) ;
#43483=LINE ( 'NONE', #22456, #11374 ) ;
#43503=DIRECTION ( 'NONE',  ( -1.000000000000000000, 0.000000000000000000, -0.000000000000000000 ) ) ;
#43516=ORIENTED_EDGE ( 'NONE', *, *, #13436, .T. ) ;
#43539=CARTESIAN_POINT ( 'NONE',  ( 939.9999999999992042, -184.9457194955397767, 62.92409052808234549 ) ) ;
#43559=ORIENTED_EDGE ( 'NONE', *, *, #31734, .T. ) ;
#43575=ORIENTED_EDGE ( 'NONE', *, *, #44398, .F. ) ;
#43689=ORIENTED_EDGE ( 'NONE', *, *, #12005, .F. ) ;
#43701=ORIENTED_EDGE ( 'NONE', *, *, #40816, .F. ) ;
#43774=DIRECTION ( 'NONE',  ( 1.000000000000000000, 2.313994520913686024E-32, 2.750100768424433609E-32 ) ) ;
#43782=LINE ( 'NONE', #23210, #22365 ) ;
#43784=ORIENTED_EDGE ( 'NONE', *, *, #30897, .F. ) ;
#43806=CARTESIAN_POINT ( 'NONE',  ( 911.9999999999992042, 219.9999999999998863, 359.9749999999999659 ) ) ;
#43897=ADVANCED_FACE ( 'NONE', ( #41285 ), #9180, .F. ) ;
#43906=CARTESIAN_POINT ( 'NONE',  ( 999.9999999999992042, -590.0000000000001137, 360.0000000000000000 ) ) ;
#43939=AXIS2_PLACEMENT_3D ( 'NONE', #30890, #23705, #44985 ) ;
#43974=ORIENTED_EDGE ( 'NONE', *, *, #43343, .F. ) ;
#43980=ORIENTED_EDGE ( 'NONE', *, *, #43330, .F. ) ;
#44000=LINE ( 'NONE', #26451, #11358 ) ;
#44059=DIRECTION ( 'NONE',  ( 1.000000000000000000, 0.000000000000000000, -0.000000000000000000 ) ) ;
#44064=AXIS2_PLACEMENT_3D ( 'NONE', #19714, #8416, #1920 ) ;
#44083=ORIENTED_EDGE ( 'NONE', *, *, #41717, .F. ) ;
#44134=DIRECTION ( 'NONE',  ( 0.000000000000000000, 1.000000000000000000, -0.000000000000000000 ) ) ;
#44180=EDGE_CURVE ( 'NONE', #29887, #23669, #1773, .T. ) ;
#44195=CIRCLE ( 'NONE', #24273, 7.999999999999896083 ) ;
#44220=DIRECTION ( 'NONE',  ( 0.000000000000000000, 0.000000000000000000, -1.000000000000000000 ) ) ;
#44222=DIRECTION ( 'NONE',  ( -0.000000000000000000, -0.000000000000000000, 1.000000000000000000 ) ) ;
#44242=CARTESIAN_POINT ( 'NONE',  ( 939.9999999999992042, 74.99999999999984368, 360.0000000000000000 ) ) ;
#44268=CARTESIAN_POINT ( 'NONE',  ( 989.9999999999992042, -431.4567479753240491, 350.0000000000000000 ) ) ;
#44306=ORIENTED_EDGE ( 'NONE', *, *, #17642, .F. ) ;
#44323=VERTEX_POINT ( 'NONE', #30886 ) ;
#44327=CARTESIAN_POINT ( 'NONE',  ( 879.9999999999992042, 239.9999999999998295, 350.0000000000000000 ) ) ;
#44388=EDGE_CURVE ( 'NONE', #8835, #2741, #9860, .T. ) ;
#44398=EDGE_CURVE ( 'NONE', #41015, #37952, #37861, .T. ) ;
#44486=VERTEX_POINT ( 'NONE', #31334 ) ;
#44521=ORIENTED_EDGE ( 'NONE', *, *, #31077, .F. ) ;
#44553=ORIENTED_EDGE ( 'NONE', *, *, #29187, .T. ) ;
#44577=LINE ( 'NONE', #37639, #29171 ) ;
#44619=CARTESIAN_POINT ( 'NONE',  ( 1820.038553321469863, -589.9999999999998863, -210.0000000000000000 ) ) ;
#44658=ORIENTED_EDGE ( 'NONE', *, *, #18752, .T. ) ;
#44663=ORIENTED_EDGE ( 'NONE', *, *, #17866, .T. ) ;
#44674=PRODUCT_DEFINITION_SHAPE ( 'NONE', 'NONE',  #42550 ) ;
#44708=PLANE ( 'NONE',  #11484 ) ;
#44712=AXIS2_PLACEMENT_3D ( 'NONE', #28662, #34500, #24721 ) ;
#44801=DIRECTION ( 'NONE',  ( 1.000000000000000000, 0.000000000000000000, 0.000000000000000000 ) ) ;
#44830=ORIENTED_EDGE ( 'NONE', *, *, #44887, .T. ) ;
#44863=DIRECTION ( 'NONE',  ( -0.000000000000000000, -0.000000000000000000, 1.000000000000000000 ) ) ;
#44879=LINE ( 'NONE', #16462, #9293 ) ;
#44887=EDGE_CURVE ( 'NONE', #31705, #16263, #14486, .T. ) ;
#44898=EDGE_LOOP ( 'NONE', ( #4952, #28807, #34672, #23442 ) ) ;
#44908=CARTESIAN_POINT ( 'NONE',  ( 919.9999999999993179, 154.9999999999998863, 360.0000000000000000 ) ) ;
#44910=EDGE_LOOP ( 'NONE', ( #43575, #36945 ) ) ;
#44962=LINE ( 'NONE', #7074, #35840 ) ;
#44981=CARTESIAN_POINT ( 'NONE',  ( 919.9999999999993179, 154.9999999999998863, -350.0000000000000000 ) ) ;
#44985=DIRECTION ( 'NONE',  ( 0.000000000000000000, -0.6594541114781790059, 0.7517448203044204691 ) ) ;
#44988=ORIENTED_EDGE ( 'NONE', *, *, #29752, .T. ) ;
#44994=DIRECTION ( 'NONE',  ( 0.000000000000000000, 1.000000000000000000, 0.000000000000000000 ) ) ;
#44999=CARTESIAN_POINT ( 'NONE',  ( 914.9999999999992042, 56.60618624968562074, 350.0000000000000000 ) ) ;
#45012=EDGE_CURVE ( 'NONE', #38205, #36984, #7667, .T. ) ;
#45140=VECTOR ( 'NONE', #9417, 1000.000000000000000 ) ;
#45182=DIRECTION ( 'NONE',  ( -1.084653538143406060E-16, 0.6594541114781790059, -0.7517448203044204691 ) ) ;
#45191=DIRECTION ( 'NONE',  ( 1.000000000000000000, 0.000000000000000000, 0.000000000000000000 ) ) ;
#45212=DIRECTION ( 'NONE',  ( 1.644774851296528363E-16, -1.000000000000000000, 0.000000000000000000 ) ) ;
#45221=ORIENTED_EDGE ( 'NONE', *, *, #16211, .T. ) ;
#45226=ORIENTED_EDGE ( 'NONE', *, *, #27795, .F. ) ;
#45259=DIRECTION ( 'NONE',  ( 1.000000000000000000, -0.000000000000000000, 0.000000000000000000 ) ) ;
#45262=VECTOR ( 'NONE', #6372, 1000.000000000000000 ) ;
#45289=EDGE_CURVE ( 'NONE', #29488, #8383, #44000, .T. ) ;
#45305=CARTESIAN_POINT ( 'NONE',  ( 879.9999999999992042, 469.9999999999998863, -350.0000000000000000 ) ) ;
#45343=EDGE_LOOP ( 'NONE', ( #13207, #13493, #17791, #34488 ) ) ;
#45345=ADVANCED_FACE ( 'NONE', ( #13055 ), #10485, .T. ) ;
#45389=VECTOR ( 'NONE', #2830, 1000.000000000000000 ) ;
#45407=VECTOR ( 'NONE', #43774, 1000.000000000000000 ) ;
#45430=FACE_OUTER_BOUND ( 'NONE', #26683, .T. ) ;
#45441=CARTESIAN_POINT ( 'NONE',  ( 939.9999999999993179, -600.0000000000001137, 350.0000000000000000 ) ) ;
#45498=VECTOR ( 'NONE', #23742, 1000.000000000000000 ) ;
#45501=VECTOR ( 'NONE', #14290, 1000.000000000000000 ) ;
#45603=CARTESIAN_POINT ( 'NONE',  ( 927.9999999999992042, 219.9999999999998863, 350.0000000000000000 ) ) ;
#45604=ORIENTED_EDGE ( 'NONE', *, *, #4995, .F. ) ;
#45607=AXIS2_PLACEMENT_3D ( 'NONE', #31189, #13643, #41829 ) ;
#45632=CARTESIAN_POINT ( 'NONE',  ( 187.1337867209877857, 62.85347435602256638, 357.4246812887967053 ) ) ;
#45663=CARTESIAN_POINT ( 'NONE',  ( 999.9999999999992042, 478.9999999999999432, -200.9999999999999432 ) ) ;
#45702=VERTEX_POINT ( 'NONE', #33344 ) ;
#45738=COLOUR_RGB('Dark Blue',0.08,0.2,0.34);
#45739=FILL_AREA_STYLE_COLOUR('',#45738);
#45740=FILL_AREA_STYLE('',(#45739));
#45741=SURFACE_STYLE_FILL_AREA(#45740);
#45742=SURFACE_SIDE_STYLE('',(#45741));
#45743=SURFACE_STYLE_USAGE(.BOTH.,#45742);
#45744=PRESENTATION_STYLE_ASSIGNMENT((#45743));
ENDSEC;
END-ISO-10303-21;
